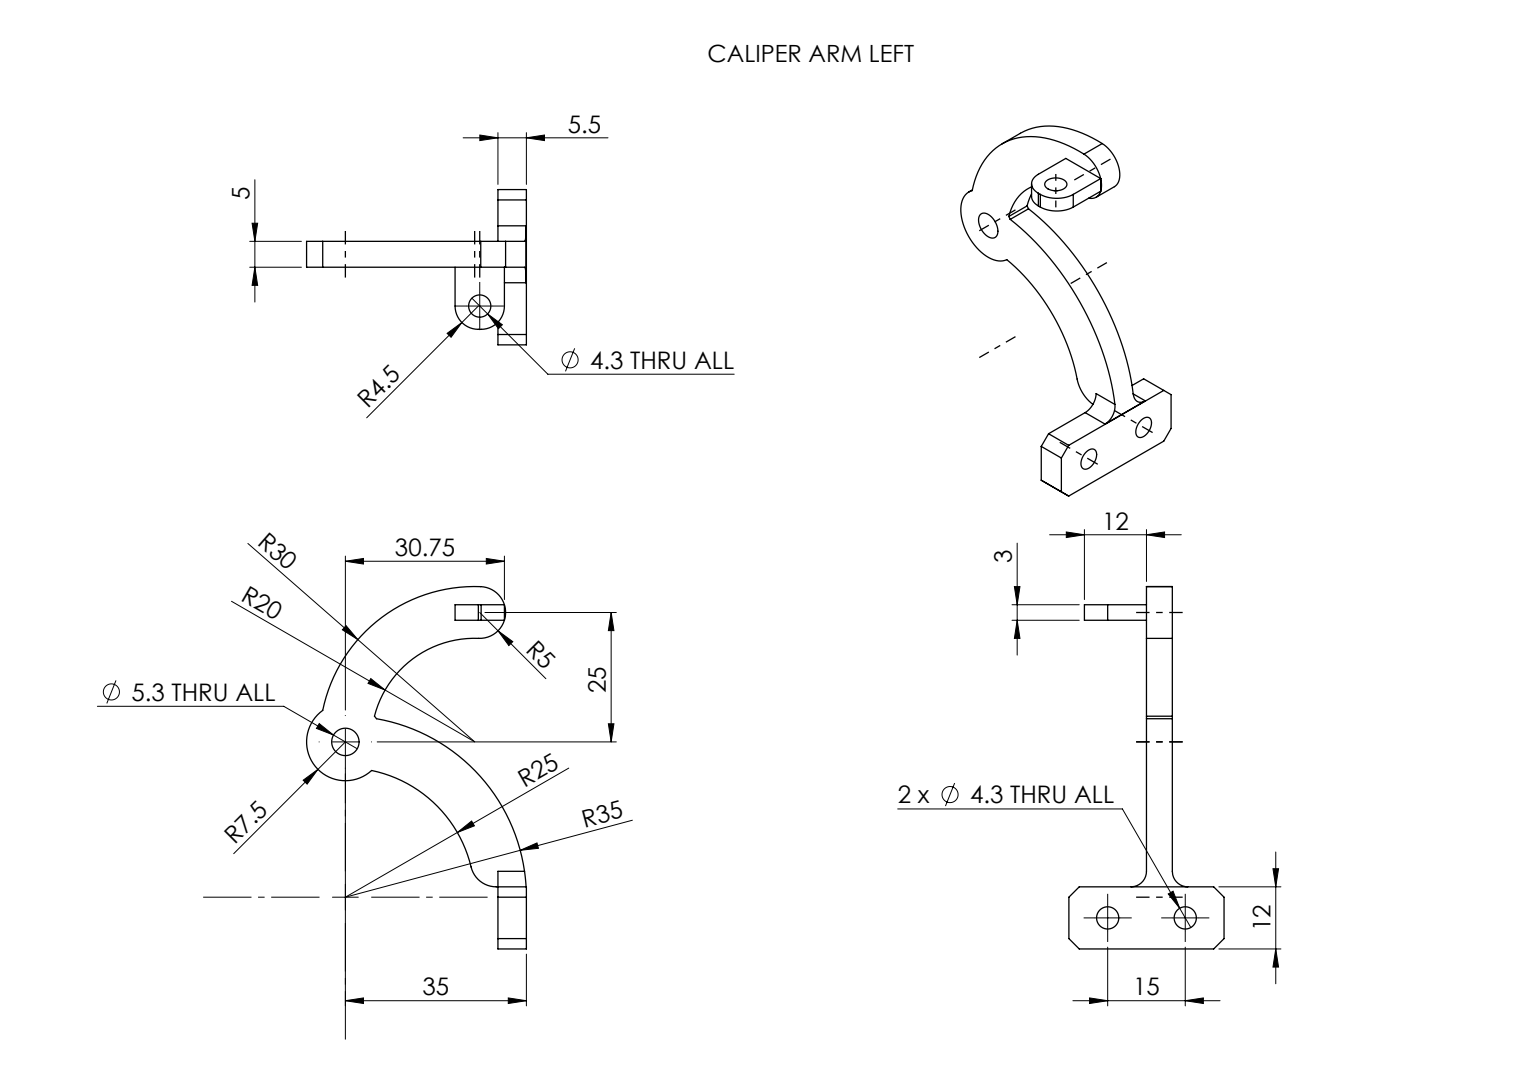
ISO-10303-21;
HEADER;
FILE_DESCRIPTION (('STEP AP214'),
    '1' );
FILE_NAME ('caliper arm left.step',
    '2026-10-08T05:45:04',
    ( '' ),
    ( '' ),
    'SwSTEP 2.0',
    'SolidWorks 2026',
    '' );
FILE_SCHEMA (( 'AUTOMOTIVE_DESIGN' ));
ENDSEC;

DATA;
#23=ADVANCED_FACE ( 'NONE', ( #9179, #3240, #3960 ), #10018, .T. ) ;
#34=CARTESIAN_POINT ( 'NONE',  ( 5.076455387921347651, 24.47916666666666075, -2.499999999999999112 ) ) ;
#40=VERTEX_POINT ( 'NONE', #10965 ) ;
#53=DIRECTION ( 'NONE',  ( 1.000000000000000000, 1.776356839400250465E-15, 0.000000000000000000 ) ) ;
#66=ORIENTED_EDGE ( 'NONE', *, *, #10280, .F. ) ;
#73=EDGE_CURVE ( 'NONE', #9208, #2549, #8067, .T. ) ;
#78=VECTOR ( 'NONE', #4837, 1000.000000000000000 ) ;
#79=DIRECTION ( 'NONE',  ( 0.000000000000000000, -1.000000000000000000, 0.000000000000000000 ) ) ;
#81=CARTESIAN_POINT ( 'NONE',  ( 29.50000000000000711, 1.387778780781445676E-14, -12.50000000000000000 ) ) ;
#86=CIRCLE ( 'NONE', #6829, 2.149999999999992362 ) ;
#90=EDGE_CURVE ( 'NONE', #5054, #1107, #1851, .T. ) ;
#96=ORIENTED_EDGE ( 'NONE', *, *, #10897, .F. ) ;
#98=EDGE_CURVE ( 'NONE', #7309, #1456, #9352, .T. ) ;
#99=FACE_OUTER_BOUND ( 'NONE', #8308, .T. ) ;
#100=AXIS2_PLACEMENT_3D ( 'NONE', #6064, #8518, #3293 ) ;
#102=CARTESIAN_POINT ( 'NONE',  ( 21.21106610644839208, 53.49999999999983658, 14.50000000000000000 ) ) ;
#108=EDGE_CURVE ( 'NONE', #2494, #2915, #8401, .T. ) ;
#112=CARTESIAN_POINT ( 'NONE',  ( 21.21106610644839208, 56.49999999999984368, 14.50000000000000000 ) ) ;
#113=EDGE_LOOP ( 'NONE', ( #698, #4129, #8999, #2220 ) ) ;
#127=DIRECTION ( 'NONE',  ( 0.000000000000000000, 0.000000000000000000, 1.000000000000000000 ) ) ;
#153=FACE_OUTER_BOUND ( 'NONE', #113, .T. ) ;
#156=ORIENTED_EDGE ( 'NONE', *, *, #2088, .F. ) ;
#176=PRESENTATION_STYLE_ASSIGNMENT (( #8567 ) ) ;
#183=VERTEX_POINT ( 'NONE', #900 ) ;
#202=CARTESIAN_POINT ( 'NONE',  ( 34.99999999999987210, -7.999999999999996447, -12.50000000000000000 ) ) ;
#208=ORIENTED_EDGE ( 'NONE', *, *, #385, .F. ) ;
#209=LINE ( 'NONE', #6940, #5064 ) ;
#217=LINE ( 'NONE', #1960, #6352 ) ;
#219=ORIENTED_EDGE ( 'NONE', *, *, #3408, .T. ) ;
#230=CARTESIAN_POINT ( 'NONE',  ( 34.99999999999987210, 2.000000000000002220, -12.50000000000000000 ) ) ;
#240=CARTESIAN_POINT ( 'NONE',  ( 6.015568632492061418, 34.47916666666664298, -2.499999999999998668 ) ) ;
#247=ORIENTED_EDGE ( 'NONE', *, *, #9284, .F. ) ;
#263=FACE_OUTER_BOUND ( 'NONE', #1330, .T. ) ;
#265=EDGE_LOOP ( 'NONE', ( #1963, #2238, #5184, #1794 ) ) ;
#277=LINE ( 'NONE', #2902, #2443 ) ;
#280=VECTOR ( 'NONE', #7293, 1000.000000000000000 ) ;
#284=CARTESIAN_POINT ( 'NONE',  ( 0.000000000000000000, 30.00000000000000000, 2.500000000000000000 ) ) ;
#289=PLANE ( 'NONE',  #436 ) ;
#290=DIRECTION ( 'NONE',  ( 0.000000000000000000, 1.000000000000000000, 0.000000000000000000 ) ) ;
#295=PLANE ( 'NONE',  #9853 ) ;
#302=EDGE_CURVE ( 'NONE', #8162, #681, #1693, .T. ) ;
#305=EDGE_CURVE ( 'NONE', #10997, #8894, #7125, .T. ) ;
#308=AXIS2_PLACEMENT_3D ( 'NONE', #6956, #4296, #9565 ) ;
#312=DIRECTION ( 'NONE',  ( -0.000000000000000000, 1.000000000000000000, -0.000000000000000000 ) ) ;
#320=CARTESIAN_POINT ( 'NONE',  ( 34.99999999999987210, -3.999999999999989786, 7.850000000000003197 ) ) ;
#322=ORIENTED_EDGE ( 'NONE', *, *, #302, .T. ) ;
#323=VECTOR ( 'NONE', #3846, 1000.000000000000114 ) ;
#355=DIRECTION ( 'NONE',  ( -6.098637220230966139E-17, 1.000000000000000000, 0.000000000000000000 ) ) ;
#371=CARTESIAN_POINT ( 'NONE',  ( 25.98076211353311749, 53.49999999999983658, 10.00000000000000178 ) ) ;
#373=AXIS2_PLACEMENT_3D ( 'NONE', #9911, #4914, #9286 ) ;
#377=ADVANCED_FACE ( 'NONE', ( #7914 ), #289, .T. ) ;
#379=ORIENTED_EDGE ( 'NONE', *, *, #4517, .F. ) ;
#381=VERTEX_POINT ( 'NONE', #2236 ) ;
#385=EDGE_CURVE ( 'NONE', #9319, #2915, #3021, .T. ) ;
#391=DIRECTION ( 'NONE',  ( 4.312387734422005941E-17, -0.7071067811865500152, 0.7071067811865451302 ) ) ;
#405=DIRECTION ( 'NONE',  ( -0.000000000000000000, -0.000000000000000000, -1.000000000000000000 ) ) ;
#410=DIRECTION ( 'NONE',  ( 1.000000000000000000, 0.000000000000000000, 0.000000000000000000 ) ) ;
#427=ORIENTED_EDGE ( 'NONE', *, *, #10489, .T. ) ;
#436=AXIS2_PLACEMENT_3D ( 'NONE', #3684, #4797, #8278 ) ;
#439=CIRCLE ( 'NONE', #9129, 7.500000000000000000 ) ;
#454=CARTESIAN_POINT ( 'NONE',  ( 24.99999259214812142, 30.01924558493218598, 2.500000000000000000 ) ) ;
#459=LINE ( 'NONE', #9638, #280 ) ;
#460=EDGE_CURVE ( 'NONE', #7106, #9208, #10799, .T. ) ;
#489=ORIENTED_EDGE ( 'NONE', *, *, #920, .T. ) ;
#492=AXIS2_PLACEMENT_3D ( 'NONE', #4378, #1817, #4149 ) ;
#498=EDGE_CURVE ( 'NONE', #8162, #10935, #5839, .T. ) ;
#500=EDGE_CURVE ( 'NONE', #2280, #1840, #8424, .T. ) ;
#505=CARTESIAN_POINT ( 'NONE',  ( 2.650000000000095834, 30.00000000000000000, -2.500000000000000000 ) ) ;
#506=ORIENTED_EDGE ( 'NONE', *, *, #5067, .T. ) ;
#524=EDGE_CURVE ( 'NONE', #2763, #4729, #7658, .T. ) ;
#529=DIRECTION ( 'NONE',  ( 1.000000000000000000, 0.000000000000000000, 0.000000000000000000 ) ) ;
#537=EDGE_LOOP ( 'NONE', ( #10892, #4237 ) ) ;
#542=ORIENTED_EDGE ( 'NONE', *, *, #9273, .T. ) ;
#558=AXIS2_PLACEMENT_3D ( 'NONE', #4552, #8823, #7936 ) ;
#565=ADVANCED_FACE ( 'NONE', ( #10231 ), #7677, .T. ) ;
#576=CARTESIAN_POINT ( 'NONE',  ( 30.75045812061784289, 53.49999999999983658, 14.50000000000000000 ) ) ;
#592=ORIENTED_EDGE ( 'NONE', *, *, #9149, .T. ) ;
#593=LINE ( 'NONE', #3109, #5602 ) ;
#606=CARTESIAN_POINT ( 'NONE',  ( 34.82492259089467979, 3.500278077966951340, -2.894288569839198022 ) ) ;
#607=LINE ( 'NONE', #3224, #5645 ) ;
#629=FACE_OUTER_BOUND ( 'NONE', #9860, .T. ) ;
#632=EDGE_CURVE ( 'NONE', #10983, #10935, #3603, .T. ) ;
#633=DIRECTION ( 'NONE',  ( 1.000000000000000000, -0.000000000000000000, -0.000000000000000000 ) ) ;
#658=CIRCLE ( 'NONE', #9718, 3.000000000000000000 ) ;
#679=ORIENTED_EDGE ( 'NONE', *, *, #9149, .F. ) ;
#681=VERTEX_POINT ( 'NONE', #6948 ) ;
#683=LINE ( 'NONE', #4766, #3461 ) ;
#684=PLANE ( 'NONE',  #6651 ) ;
#698=ORIENTED_EDGE ( 'NONE', *, *, #108, .F. ) ;
#701=PLANE ( 'NONE',  #10710 ) ;
#712=AXIS2_PLACEMENT_3D ( 'NONE', #9244, #9413, #4259 ) ;
#731=DIRECTION ( 'NONE',  ( -0.000000000000000000, 1.000000000000000000, -0.000000000000000000 ) ) ;
#738=DIRECTION ( 'NONE',  ( -0.000000000000000000, -0.000000000000000000, -1.000000000000000000 ) ) ;
#748=ORIENTED_EDGE ( 'NONE', *, *, #5542, .F. ) ;
#750=VERTEX_POINT ( 'NONE', #7844 ) ;
#758=DIRECTION ( 'NONE',  ( -1.000000000000000000, 0.000000000000000000, 0.000000000000000000 ) ) ;
#776=CARTESIAN_POINT ( 'NONE',  ( 29.50000000000000711, -3.999999999999989786, -2.850000000000007194 ) ) ;
#786=CIRCLE ( 'NONE', #10023, 2.649999999999992362 ) ;
#788=VECTOR ( 'NONE', #2505, 1000.000000000000000 ) ;
#796=CARTESIAN_POINT ( 'NONE',  ( 25.71106610644839208, 53.49999999999983658, 14.50000000000000000 ) ) ;
#823=EDGE_CURVE ( 'NONE', #8525, #1015, #3146, .T. ) ;
#826=CYLINDRICAL_SURFACE ( 'NONE', #6009, 7.500000000000000000 ) ;
#830=CARTESIAN_POINT ( 'NONE',  ( 6.098637220230963427E-16, -10.00000000000000000, 0.000000000000000000 ) ) ;
#832=ORIENTED_EDGE ( 'NONE', *, *, #10941, .F. ) ;
#841=AXIS2_PLACEMENT_3D ( 'NONE', #5509, #10615, #4675 ) ;
#842=COLOUR_RGB ( '', 0.72549020, 0.75294118, 0.79215686) ;
#847=DIRECTION ( 'NONE',  ( -1.000000000000000000, -6.098637220230963674E-17, 0.000000000000000000 ) ) ;
#852=CYLINDRICAL_SURFACE ( 'NONE', #1893, 2.149999999999988809 ) ;
#858=CARTESIAN_POINT ( 'NONE',  ( 34.90196196521935690, 2.620161469061431880, 3.662783066803843468 ) ) ;
#861=CARTESIAN_POINT ( 'NONE',  ( 34.99999999999987210, -9.999999999999998224, -10.50000000000001243 ) ) ;
#867=EDGE_CURVE ( 'NONE', #9108, #1634, #6971, .T. ) ;
#874=VERTEX_POINT ( 'NONE', #8674 ) ;
#891=ORIENTED_EDGE ( 'NONE', *, *, #7285, .T. ) ;
#900=CARTESIAN_POINT ( 'NONE',  ( 25.98076211353311749, 56.49999999999984368, 7.850000000000009415 ) ) ;
#905=EDGE_CURVE ( 'NONE', #7610, #10564, #3067, .T. ) ;
#916=EDGE_LOOP ( 'NONE', ( #9339, #3984, #219, #3158 ) ) ;
#917=CARTESIAN_POINT ( 'NONE',  ( 29.50000000000000711, -7.999999999999996447, -12.50000000000000000 ) ) ;
#918=CARTESIAN_POINT ( 'NONE',  ( 34.99999999999987210, 2.000000000000002220, -10.49999999999999822 ) ) ;
#920=EDGE_CURVE ( 'NONE', #7348, #750, #2720, .T. ) ;
#924=DIRECTION ( 'NONE',  ( 1.000000000000000000, -0.000000000000000000, -0.000000000000000000 ) ) ;
#926=VECTOR ( 'NONE', #5218, 1000.000000000000114 ) ;
#934=FACE_OUTER_BOUND ( 'NONE', #7050, .T. ) ;
#935=DIRECTION ( 'NONE',  ( -0.000000000000000000, -0.000000000000000000, -1.000000000000000000 ) ) ;
#953=EDGE_CURVE ( 'NONE', #1015, #6697, #6053, .T. ) ;
#955=CARTESIAN_POINT ( 'NONE',  ( -1.219727444046192735E-16, 2.000000000000000000, -10.49999999999999822 ) ) ;
#972=FILL_AREA_STYLE ('',( #1601 ) ) ;
#973=AXIS2_PLACEMENT_3D ( 'NONE', #3761, #312, #4606 ) ;
#975=VECTOR ( 'NONE', #847, 1000.000000000000000 ) ;
#983=CARTESIAN_POINT ( 'NONE',  ( 34.99999999999987210, 2.000000000000002220, 15.49999999999999645 ) ) ;
#992=AXIS2_PLACEMENT_3D ( 'NONE', #9238, #4978, #5147 ) ;
#1003=ORIENTED_EDGE ( 'NONE', *, *, #8256, .T. ) ;
#1012=DIRECTION ( 'NONE',  ( 1.000000000000000000, -2.212882687011047826E-16, 0.000000000000000000 ) ) ;
#1015=VERTEX_POINT ( 'NONE', #6180 ) ;
#1016=LINE ( 'NONE', #10524, #1355 ) ;
#1018=AXIS2_PLACEMENT_3D ( 'NONE', #830, #6007, #6951 ) ;
#1037=DIRECTION ( 'NONE',  ( 2.212882687011047826E-16, 1.000000000000000000, -0.000000000000000000 ) ) ;
#1043=CARTESIAN_POINT ( 'NONE',  ( 34.99999999999987210, 1.431146867680865853E-14, -12.50000000000000000 ) ) ;
#1044=PRODUCT_CONTEXT ( 'NONE', #7789, 'mechanical' ) ;
#1053=ORIENTED_EDGE ( 'NONE', *, *, #9284, .T. ) ;
#1055=ORIENTED_EDGE ( 'NONE', *, *, #8721, .T. ) ;
#1057=ORIENTED_EDGE ( 'NONE', *, *, #6360, .T. ) ;
#1076=LINE ( 'NONE', #10587, #10450 ) ;
#1083=CARTESIAN_POINT ( 'NONE',  ( -3.049318610115482207E-16, 5.000000000000000000, 5.500000000000000000 ) ) ;
#1085=FACE_OUTER_BOUND ( 'NONE', #3210, .T. ) ;
#1092=EDGE_CURVE ( 'NONE', #1254, #8525, #5107, .T. ) ;
#1093=VERTEX_POINT ( 'NONE', #34 ) ;
#1094=CARTESIAN_POINT ( 'NONE',  ( 30.75045812061784289, 53.49999999999983658, 2.500000000000000000 ) ) ;
#1098=DIRECTION ( 'NONE',  ( 0.000000000000000000, 1.000000000000000000, 0.000000000000000000 ) ) ;
#1104=ADVANCED_FACE ( 'NONE', ( #153 ), #7714, .F. ) ;
#1107=VERTEX_POINT ( 'NONE', #3319 ) ;
#1108=DIRECTION ( 'NONE',  ( 6.098637220230963674E-17, -1.000000000000000000, 0.000000000000000000 ) ) ;
#1111=VECTOR ( 'NONE', #4090, 1000.000000000000000 ) ;
#1114=( LENGTH_UNIT ( ) NAMED_UNIT ( * ) SI_UNIT ( .MILLI., .METRE. ) );
#1120=DIRECTION ( 'NONE',  ( 0.000000000000000000, 0.000000000000000000, -1.000000000000000000 ) ) ;
#1123=ORIENTED_EDGE ( 'NONE', *, *, #4241, .F. ) ;
#1132=CARTESIAN_POINT ( 'NONE',  ( 34.94281041931228771, 2.000000000000002220, 2.500000000000000000 ) ) ;
#1133=CIRCLE ( 'NONE', #8225, 4.999999999999997335 ) ;
#1134=ORIENTED_EDGE ( 'NONE', *, *, #5268, .F. ) ;
#1141=CYLINDRICAL_SURFACE ( 'NONE', #973, 2.149999999999988809 ) ;
#1143=DIRECTION ( 'NONE',  ( -0.000000000000000000, 1.000000000000000000, -0.000000000000000000 ) ) ;
#1145=AXIS2_PLACEMENT_3D ( 'NONE', #6201, #9587, #410 ) ;
#1149=CIRCLE ( 'NONE', #5763, 2.149999999999988809 ) ;
#1154=CARTESIAN_POINT ( 'NONE',  ( 34.99999999999987210, 1.431146867680865853E-14, 17.49999999999999645 ) ) ;
#1156=DIRECTION ( 'NONE',  ( 0.000000000000000000, -1.000000000000000000, 0.000000000000000000 ) ) ;
#1163=ORIENTED_EDGE ( 'NONE', *, *, #6957, .T. ) ;
#1167=VECTOR ( 'NONE', #6619, 1000.000000000000000 ) ;
#1179=EDGE_CURVE ( 'NONE', #681, #3312, #8596, .T. ) ;
#1180=ORIENTED_EDGE ( 'NONE', *, *, #8476, .T. ) ;
#1202=EDGE_CURVE ( 'NONE', #6168, #6073, #6594, .T. ) ;
#1206=CARTESIAN_POINT ( 'NONE',  ( 34.99999999999987210, -9.999999999999998224, 15.49999999999998934 ) ) ;
#1207=VECTOR ( 'NONE', #9723, 1000.000000000000000 ) ;
#1209=LINE ( 'NONE', #7937, #5883 ) ;
#1224=ORIENTED_EDGE ( 'NONE', *, *, #5136, .F. ) ;
#1237=CARTESIAN_POINT ( 'NONE',  ( 21.21106610644839208, 53.49999999999983658, 14.50000000000000000 ) ) ;
#1253=CARTESIAN_POINT ( 'NONE',  ( 29.50000000000000711, -3.999999999999989786, 9.999999999999998224 ) ) ;
#1254=VERTEX_POINT ( 'NONE', #983 ) ;
#1281=ORIENTED_EDGE ( 'NONE', *, *, #1179, .T. ) ;
#1295=EDGE_LOOP ( 'NONE', ( #8009, #4620, #5332, #9406 ) ) ;
#1298=CYLINDRICAL_SURFACE ( 'NONE', #5272, 2.649999999999991029 ) ;
#1305=CARTESIAN_POINT ( 'NONE',  ( 21.21106610644839208, 56.49999999999984368, 14.50000000000000000 ) ) ;
#1307=LINE ( 'NONE', #3915, #5108 ) ;
#1309=CYLINDRICAL_SURFACE ( 'NONE', #5601, 3.000000000000000000 ) ;
#1314=VECTOR ( 'NONE', #2944, 1000.000000000000000 ) ;
#1315=DIRECTION ( 'NONE',  ( 0.000000000000000000, -1.000000000000000000, 0.000000000000000000 ) ) ;
#1323=ORIENTED_EDGE ( 'NONE', *, *, #3560, .T. ) ;
#1324=EDGE_CURVE ( 'NONE', #4849, #2261, #6962, .T. ) ;
#1325=CARTESIAN_POINT ( 'NONE',  ( 34.94281041931228771, 5.000000000000001776, 2.500000000000000000 ) ) ;
#1327=VECTOR ( 'NONE', #7145, 1000.000000000000000 ) ;
#1330=EDGE_LOOP ( 'NONE', ( #5656, #4328, #8187, #2492 ) ) ;
#1336=AXIS2_PLACEMENT_3D ( 'NONE', #5007, #8382, #758 ) ;
#1337=ORIENTED_EDGE ( 'NONE', *, *, #10941, .T. ) ;
#1354=EDGE_CURVE ( 'NONE', #183, #9110, #8369, .T. ) ;
#1355=VECTOR ( 'NONE', #9627, 1000.000000000000000 ) ;
#1373=LINE ( 'NONE', #576, #5611 ) ;
#1375=PRODUCT_DEFINITION ( 'UNKNOWN', '', #7225, #8335 ) ;
#1376=CIRCLE ( 'NONE', #5462, 2.149999999999992362 ) ;
#1384=VECTOR ( 'NONE', #5130, 1000.000000000000000 ) ;
#1402=EDGE_CURVE ( 'NONE', #6697, #1254, #6987, .T. ) ;
#1404=CARTESIAN_POINT ( 'NONE',  ( 34.94281041931228771, 2.000000000000002665, -5.301324476612966130 ) ) ;
#1413=CARTESIAN_POINT ( 'NONE',  ( 21.21106610644839208, 56.49999999999984368, 2.500000000000000000 ) ) ;
#1415=DIRECTION ( 'NONE',  ( -0.000000000000000000, 0.000000000000000000, 1.000000000000000000 ) ) ;
#1436=UNCERTAINTY_MEASURE_WITH_UNIT (LENGTH_MEASURE( 1.000000000000000082E-05 ), #6013, 'distance_accuracy_value', 'NONE');
#1437=VERTEX_POINT ( 'NONE', #7881 ) ;
#1445=ORIENTED_EDGE ( 'NONE', *, *, #6596, .F. ) ;
#1449=EDGE_CURVE ( 'NONE', #7957, #3879, #3596, .T. ) ;
#1453=DIRECTION ( 'NONE',  ( 1.000000000000000000, -0.000000000000000000, -0.000000000000000000 ) ) ;
#1456=VERTEX_POINT ( 'NONE', #1206 ) ;
#1462=CARTESIAN_POINT ( 'NONE',  ( 34.64101615137754919, 5.000000000000002665, 2.500000000000000000 ) ) ;
#1469=ORIENTED_EDGE ( 'NONE', *, *, #9598, .F. ) ;
#1471=LINE ( 'NONE', #10802, #4745 ) ;
#1493=VERTEX_POINT ( 'NONE', #5806 ) ;
#1503=CARTESIAN_POINT ( 'NONE',  ( 34.69578914996070296, 4.608685395970379517, -2.519144107514304398 ) ) ;
#1510=VECTOR ( 'NONE', #4752, 1000.000000000000000 ) ;
#1526=DIRECTION ( 'NONE',  ( 1.000000000000000000, 0.000000000000000000, 0.000000000000000000 ) ) ;
#1532=CARTESIAN_POINT ( 'NONE',  ( 5.621179405865835754, 34.96511249490581008, 2.500000000000000000 ) ) ;
#1554=AXIS2_PLACEMENT_3D ( 'NONE', #2026, #4533, #9634 ) ;
#1563=ORIENTED_EDGE ( 'NONE', *, *, #6544, .T. ) ;
#1571=CARTESIAN_POINT ( 'NONE',  ( 29.50000000000000711, 2.000000000000001776, 2.500000000000000444 ) ) ;
#1575=EDGE_LOOP ( 'NONE', ( #5448, #9550, #1180, #4570 ) ) ;
#1584=CARTESIAN_POINT ( 'NONE',  ( 34.92403196580097813, 2.306010598194981664, 4.165547504151214220 ) ) ;
#1592=LINE ( 'NONE', #10985, #9194 ) ;
#1601=FILL_AREA_STYLE_COLOUR ( '', #8306 ) ;
#1603=EDGE_LOOP ( 'NONE', ( #4104, #1053, #1842, #4564 ) ) ;
#1607=EDGE_LOOP ( 'NONE', ( #4800, #10163, #96, #4089, #10341, #4390, #748, #2683, #7548, #10701, #1055 ) ) ;
#1610=CYLINDRICAL_SURFACE ( 'NONE', #1336, 4.999999999999997335 ) ;
#1619=ORIENTED_EDGE ( 'NONE', *, *, #823, .T. ) ;
#1632=DIRECTION ( 'NONE',  ( 4.312387734421997929E-17, -0.7071067811865487940, -0.7071067811865463515 ) ) ;
#1634=VERTEX_POINT ( 'NONE', #6749 ) ;
#1635=ORIENTED_EDGE ( 'NONE', *, *, #7169, .F. ) ;
#1648=DIRECTION ( 'NONE',  ( 1.000000000000000000, -9.251858538542971828E-16, 0.000000000000000000 ) ) ;
#1656=ORIENTED_EDGE ( 'NONE', *, *, #3408, .F. ) ;
#1657=DIRECTION ( 'NONE',  ( 0.000000000000000000, -1.000000000000000000, 0.000000000000000000 ) ) ;
#1662=VERTEX_POINT ( 'NONE', #796 ) ;
#1664=DIRECTION ( 'NONE',  ( -1.000000000000000000, -6.098637220230963674E-17, 0.000000000000000000 ) ) ;
#1682=VECTOR ( 'NONE', #1012, 1000.000000000000000 ) ;
#1693=CIRCLE ( 'NONE', #7367, 4.500000000000000000 ) ;
#1702=VECTOR ( 'NONE', #2138, 1000.000000000000000 ) ;
#1718=CARTESIAN_POINT ( 'NONE',  ( 0.000000000000000000, 30.00000000000000000, -2.499999999999998668 ) ) ;
#1753=ADVANCED_FACE ( 'NONE', ( #4316 ), #5917, .T. ) ;
#1765=DIRECTION ( 'NONE',  ( -1.000000000000000000, -6.098637220230963674E-17, 0.000000000000000000 ) ) ;
#1766=ORIENTED_EDGE ( 'NONE', *, *, #2279, .F. ) ;
#1767=LINE ( 'NONE', #917, #7339 ) ;
#1782=FACE_OUTER_BOUND ( 'NONE', #1603, .T. ) ;
#1794=ORIENTED_EDGE ( 'NONE', *, *, #3531, .F. ) ;
#1805=EDGE_CURVE ( 'NONE', #10564, #183, #7190, .T. ) ;
#1815=LINE ( 'NONE', #7089, #3829 ) ;
#1816=ORIENTED_EDGE ( 'NONE', *, *, #10153, .F. ) ;
#1817=DIRECTION ( 'NONE',  ( 0.000000000000000000, -0.000000000000000000, -1.000000000000000000 ) ) ;
#1823=CARTESIAN_POINT ( 'NONE',  ( 30.75045812061784289, 56.49999999999984368, 14.50000000000000000 ) ) ;
#1832=EDGE_CURVE ( 'NONE', #7103, #7090, #1076, .T. ) ;
#1833=DIRECTION ( 'NONE',  ( 0.000000000000000000, 0.000000000000000000, -1.000000000000000000 ) ) ;
#1835=CARTESIAN_POINT ( 'NONE',  ( 34.64101615137754919, 5.000000000000002665, -2.500000000000000000 ) ) ;
#1840=VERTEX_POINT ( 'NONE', #8643 ) ;
#1841=FACE_OUTER_BOUND ( 'NONE', #10523, .T. ) ;
#1842=ORIENTED_EDGE ( 'NONE', *, *, #524, .F. ) ;
#1851=LINE ( 'NONE', #955, #975 ) ;
#1852=DIRECTION ( 'NONE',  ( 0.000000000000000000, 1.000000000000000000, 0.000000000000000000 ) ) ;
#1855=ORIENTED_EDGE ( 'NONE', *, *, #7793, .F. ) ;
#1869=( NAMED_UNIT ( * ) SI_UNIT ( $, .STERADIAN. ) SOLID_ANGLE_UNIT ( ) );
#1872=VECTOR ( 'NONE', #7281, 1000.000000000000000 ) ;
#1885=ORIENTED_EDGE ( 'NONE', *, *, #5967, .F. ) ;
#1892=PLANE ( 'NONE',  #4534 ) ;
#1893=AXIS2_PLACEMENT_3D ( 'NONE', #10249, #731, #2411 ) ;
#1909=FILL_AREA_STYLE ('',( #10293 ) ) ;
#1913=CARTESIAN_POINT ( 'NONE',  ( 29.50000000000000711, -7.999999999999996447, -12.50000000000000000 ) ) ;
#1919=PLANE ( 'NONE',  #4194 ) ;
#1933=CIRCLE ( 'NONE', #492, 20.00000000000000355 ) ;
#1937=ADVANCED_FACE ( 'NONE', ( #9856 ), #8080, .T. ) ;
#1951=VERTEX_POINT ( 'NONE', #1413 ) ;
#1954=ADVANCED_FACE ( 'NONE', ( #4806 ), #826, .T. ) ;
#1956=DIRECTION ( 'NONE',  ( 0.000000000000000000, 0.000000000000000000, 1.000000000000000000 ) ) ;
#1960=CARTESIAN_POINT ( 'NONE',  ( 29.50000000000000711, 2.000000000000001776, -12.50000000000000000 ) ) ;
#1963=ORIENTED_EDGE ( 'NONE', *, *, #2382, .F. ) ;
#1973=FACE_OUTER_BOUND ( 'NONE', #8882, .T. ) ;
#1993=ORIENTED_EDGE ( 'NONE', *, *, #1324, .T. ) ;
#1997=DIRECTION ( 'NONE',  ( 1.000000000000000000, -0.000000000000000000, -0.000000000000000000 ) ) ;
#2018=PLANE ( 'NONE',  #10066 ) ;
#2023=LINE ( 'NONE', #9746, #1702 ) ;
#2026=CARTESIAN_POINT ( 'NONE',  ( 0.000000000000000000, 0.000000000000000000, -2.500000000000000000 ) ) ;
#2033=CARTESIAN_POINT ( 'NONE',  ( 34.99999999999987210, 2.000000000000002220, 17.49999999999999645 ) ) ;
#2045=ORIENTED_EDGE ( 'NONE', *, *, #4707, .F. ) ;
#2056=EDGE_CURVE ( 'NONE', #3381, #7103, #2651, .T. ) ;
#2088=EDGE_CURVE ( 'NONE', #1662, #10997, #5832, .T. ) ;
#2098=PLANE ( 'NONE',  #3491 ) ;
#2103=PRODUCT_DEFINITION_SHAPE ( 'NONE', 'NONE',  #1375 ) ;
#2114=VECTOR ( 'NONE', #6232, 1000.000000000000000 ) ;
#2116=CARTESIAN_POINT ( 'NONE',  ( 25.71106610644839208, 0.000000000000000000, 14.50000000000000000 ) ) ;
#2138=DIRECTION ( 'NONE',  ( -1.000000000000000000, -6.098637220230963674E-17, -0.000000000000000000 ) ) ;
#2139=DIRECTION ( 'NONE',  ( 1.000000000000000000, 0.000000000000000000, 0.000000000000000000 ) ) ;
#2150=CARTESIAN_POINT ( 'NONE',  ( 0.000000000000000000, 0.000000000000000000, 2.500000000000000000 ) ) ;
#2169=DIRECTION ( 'NONE',  ( 1.000000000000000000, 0.000000000000000000, 0.000000000000000000 ) ) ;
#2178=AXIS2_PLACEMENT_3D ( 'NONE', #9556, #8722, #1956 ) ;
#2179=CARTESIAN_POINT ( 'NONE',  ( 34.91794119163850496, 2.397787035234373310, -3.994322637888108485 ) ) ;
#2181=ORIENTED_EDGE ( 'NONE', *, *, #2382, .T. ) ;
#2182=ORIENTED_EDGE ( 'NONE', *, *, #6710, .F. ) ;
#2189=DIRECTION ( 'NONE',  ( 0.000000000000000000, -1.000000000000000000, 0.000000000000000000 ) ) ;
#2194=DIRECTION ( 'NONE',  ( -0.000000000000000000, -1.000000000000000000, -0.000000000000000000 ) ) ;
#2196=CARTESIAN_POINT ( 'NONE',  ( 29.50000000000000711, 2.000000000000001776, 5.500000000000001776 ) ) ;
#2200=VECTOR ( 'NONE', #6936, 1000.000000000000000 ) ;
#2204=ORIENTED_EDGE ( 'NONE', *, *, #6466, .T. ) ;
#2211=ADVANCED_FACE ( 'NONE', ( #10845 ), #8343, .F. ) ;
#2218=EDGE_CURVE ( 'NONE', #5054, #1254, #6733, .T. ) ;
#2220=ORIENTED_EDGE ( 'NONE', *, *, #3035, .F. ) ;
#2236=CARTESIAN_POINT ( 'NONE',  ( 34.94281041931228771, 2.000000000000002220, 5.500000000000000000 ) ) ;
#2238=ORIENTED_EDGE ( 'NONE', *, *, #8447, .F. ) ;
#2250=EDGE_LOOP ( 'NONE', ( #9722, #6708, #2722, #208, #9563, #2628, #427, #9652, #10160, #1123, #3401, #7607, #9046, #2783, #2836 ) ) ;
#2261=VERTEX_POINT ( 'NONE', #776 ) ;
#2274=ORIENTED_EDGE ( 'NONE', *, *, #6710, .T. ) ;
#2279=EDGE_CURVE ( 'NONE', #6762, #2549, #5527, .T. ) ;
#2280=VERTEX_POINT ( 'NONE', #3294 ) ;
#2283=LINE ( 'NONE', #2440, #78 ) ;
#2332=CARTESIAN_POINT ( 'NONE',  ( 29.50000000000000711, 1.387778780781445676E-14, 17.49999999999999645 ) ) ;
#2336=CARTESIAN_POINT ( 'NONE',  ( 34.76713615931384993, 4.034733667027952997, -2.652855901285304796 ) ) ;
#2344=CARTESIAN_POINT ( 'NONE',  ( 34.74418829745650328, 4.228279689541293962, 2.594445730714923126 ) ) ;
#2356=FACE_OUTER_BOUND ( 'NONE', #2946, .T. ) ;
#2363=ORIENTED_EDGE ( 'NONE', *, *, #4819, .F. ) ;
#2382=EDGE_CURVE ( 'NONE', #6022, #381, #7696, .T. ) ;
#2385=DIRECTION ( 'NONE',  ( 1.000000000000000000, 0.000000000000000000, 0.000000000000000000 ) ) ;
#2392=VECTOR ( 'NONE', #1632, 1000.000000000000000 ) ;
#2410=EDGE_LOOP ( 'NONE', ( #2733, #5468, #10851, #4676 ) ) ;
#2411=DIRECTION ( 'NONE',  ( 0.000000000000000000, 0.000000000000000000, 1.000000000000000000 ) ) ;
#2412=AXIS2_PLACEMENT_3D ( 'NONE', #9025, #1415, #4808 ) ;
#2419=CARTESIAN_POINT ( 'NONE',  ( 34.94281041931228771, 2.000000000000002220, 5.500000000000000000 ) ) ;
#2435=ADVANCED_FACE ( 'NONE', ( #10143 ), #10916, .F. ) ;
#2440=CARTESIAN_POINT ( 'NONE',  ( 21.21106610644839208, 53.49999999999983658, 14.50000000000000000 ) ) ;
#2443=VECTOR ( 'NONE', #8893, 1000.000000000000000 ) ;
#2445=AXIS2_PLACEMENT_3D ( 'NONE', #8555, #4162, #2385 ) ;
#2452=MECHANICAL_DESIGN_GEOMETRIC_PRESENTATION_REPRESENTATION('',(#4953),#5300);
#2456=LINE ( 'NONE', #505, #5292 ) ;
#2492=ORIENTED_EDGE ( 'NONE', *, *, #6360, .F. ) ;
#2494=VERTEX_POINT ( 'NONE', #4136 ) ;
#2497=ORIENTED_EDGE ( 'NONE', *, *, #5677, .F. ) ;
#2505=DIRECTION ( 'NONE',  ( -1.000000000000000000, -0.000000000000000000, -0.000000000000000000 ) ) ;
#2529=UNCERTAINTY_MEASURE_WITH_UNIT (LENGTH_MEASURE( 1.000000000000000082E-05 ), #1114, 'distance_accuracy_value', 'NONE');
#2542=EDGE_CURVE ( 'NONE', #7103, #3195, #2874, .T. ) ;
#2549=VERTEX_POINT ( 'NONE', #240 ) ;
#2552=ORIENTED_EDGE ( 'NONE', *, *, #73, .T. ) ;
#2556=DIRECTION ( 'NONE',  ( 0.000000000000000000, 0.000000000000000000, 1.000000000000000000 ) ) ;
#2584=ORIENTED_EDGE ( 'NONE', *, *, #1092, .F. ) ;
#2586=ORIENTED_EDGE ( 'NONE', *, *, #90, .T. ) ;
#2588=VECTOR ( 'NONE', #2556, 1000.000000000000000 ) ;
#2624=CARTESIAN_POINT ( 'NONE',  ( 1.047444401652940007E-13, 30.00000000000000000, -2.500000000000000000 ) ) ;
#2628=ORIENTED_EDGE ( 'NONE', *, *, #8772, .T. ) ;
#2644=DIRECTION ( 'NONE',  ( -0.000000000000000000, 0.000000000000000000, 1.000000000000000000 ) ) ;
#2651=CIRCLE ( 'NONE', #8852, 20.00000000000000355 ) ;
#2670=DIRECTION ( 'NONE',  ( 1.000000000000000000, 0.000000000000000000, 0.000000000000000000 ) ) ;
#2680=CARTESIAN_POINT ( 'NONE',  ( 24.99999259214812142, 30.01924558493218598, 2.500000000000000000 ) ) ;
#2683=ORIENTED_EDGE ( 'NONE', *, *, #2279, .T. ) ;
#2710=ORIENTED_EDGE ( 'NONE', *, *, #6636, .F. ) ;
#2714=AXIS2_PLACEMENT_3D ( 'NONE', #3816, #1143, #2883 ) ;
#2718=CARTESIAN_POINT ( 'NONE',  ( 34.99999999999987210, -3.999999999999989786, -4.999999999999999112 ) ) ;
#2720=CIRCLE ( 'NONE', #6422, 2.649999999999992362 ) ;
#2722=ORIENTED_EDGE ( 'NONE', *, *, #108, .T. ) ;
#2733=ORIENTED_EDGE ( 'NONE', *, *, #1179, .F. ) ;
#2755=CIRCLE ( 'NONE', #1145, 35.00000000000000000 ) ;
#2763=VERTEX_POINT ( 'NONE', #3076 ) ;
#2770=CIRCLE ( 'NONE', #7047, 30.00000000000000000 ) ;
#2774=DIRECTION ( 'NONE',  ( -0.000000000000000000, 0.000000000000000000, 1.000000000000000000 ) ) ;
#2778=VECTOR ( 'NONE', #9473, 1000.000000000000000 ) ;
#2783=ORIENTED_EDGE ( 'NONE', *, *, #5002, .F. ) ;
#2789=CARTESIAN_POINT ( 'NONE',  ( 25.98076211353311749, 53.49999999999983658, 10.00000000000000178 ) ) ;
#2800=LINE ( 'NONE', #9618, #9007 ) ;
#2804=CARTESIAN_POINT ( 'NONE',  ( 29.17190429162964094, 2.000000000000001776, 17.50099999999999767 ) ) ;
#2806=VECTOR ( 'NONE', #8913, 1000.000000000000000 ) ;
#2825=AXIS2_PLACEMENT_3D ( 'NONE', #1083, #7823, #355 ) ;
#2829=CARTESIAN_POINT ( 'NONE',  ( -1.219727444046192735E-16, 2.000000000000000000, 0.000000000000000000 ) ) ;
#2836=ORIENTED_EDGE ( 'NONE', *, *, #8107, .T. ) ;
#2839=DIRECTION ( 'NONE',  ( 4.312387734421975743E-17, -0.7071067811865451302, -0.7071067811865500152 ) ) ;
#2840=ADVANCED_BREP_SHAPE_REPRESENTATION ( '', ( #5541, #308 ), #10083 ) ;
#2857=CARTESIAN_POINT ( 'NONE',  ( 29.17190429162964094, 7.000000000000002665, -2.500000000000000000 ) ) ;
#2865=FACE_OUTER_BOUND ( 'NONE', #2250, .T. ) ;
#2874=CIRCLE ( 'NONE', #712, 4.999999999999997335 ) ;
#2883=DIRECTION ( 'NONE',  ( 0.000000000000000000, 0.000000000000000000, 1.000000000000000000 ) ) ;
#2885=ORIENTED_EDGE ( 'NONE', *, *, #953, .T. ) ;
#2894=DIRECTION ( 'NONE',  ( 1.000000000000000000, 6.098637220230963674E-17, -0.000000000000000000 ) ) ;
#2902=CARTESIAN_POINT ( 'NONE',  ( 26.25045812061784289, 0.000000000000000000, 14.50000000000000000 ) ) ;
#2905=ORIENTED_EDGE ( 'NONE', *, *, #8772, .F. ) ;
#2914=DIRECTION ( 'NONE',  ( 1.000000000000000000, 6.098637220230963674E-17, 0.000000000000000000 ) ) ;
#2915=VERTEX_POINT ( 'NONE', #1571 ) ;
#2916=EDGE_LOOP ( 'NONE', ( #2274, #7235, #8984, #4264, #6768, #2885, #7111, #10354, #3084, #7563, #6085, #1163, #1003, #4364 ) ) ;
#2918=DIRECTION ( 'NONE',  ( 1.000000000000000000, 0.000000000000000000, 0.000000000000000000 ) ) ;
#2930=LINE ( 'NONE', #2033, #4032 ) ;
#2935=AXIS2_PLACEMENT_3D ( 'NONE', #1718, #9488, #8378 ) ;
#2944=DIRECTION ( 'NONE',  ( 0.000000000000000000, 1.000000000000000000, 0.000000000000000000 ) ) ;
#2946=EDGE_LOOP ( 'NONE', ( #2552, #5823, #2905, #2181, #1323, #5683 ) ) ;
#2988=AXIS2_PLACEMENT_3D ( 'NONE', #10784, #1453, #5680 ) ;
#3000=EDGE_LOOP ( 'NONE', ( #9977, #1656, #1469, #5840, #10769, #4986 ) ) ;
#3003=AXIS2_PLACEMENT_3D ( 'NONE', #9371, #3431, #6806 ) ;
#3016=SHAPE_REPRESENTATION ( 'caliper arm left', ( #308 ), #10083 ) ;
#3021=LINE ( 'NONE', #10001, #1872 ) ;
#3024=VERTEX_POINT ( 'NONE', #1913 ) ;
#3030=CARTESIAN_POINT ( 'NONE',  ( 0.000000000000000000, 30.00000000000000000, -23.71320343559643007 ) ) ;
#3035=EDGE_CURVE ( 'NONE', #2915, #40, #1209, .T. ) ;
#3037=CARTESIAN_POINT ( 'NONE',  ( 30.75045812061784289, 53.49999999999983658, 10.00000000000000178 ) ) ;
#3063=AXIS2_PLACEMENT_3D ( 'NONE', #2718, #924, #6874 ) ;
#3067=CIRCLE ( 'NONE', #6078, 2.149999999999988809 ) ;
#3068=CARTESIAN_POINT ( 'NONE',  ( 34.94281041931228771, 2.000000000000002220, -5.500000000000000000 ) ) ;
#3069=DIRECTION ( 'NONE',  ( 1.000000000000000000, 6.098637220230963674E-17, 0.000000000000000000 ) ) ;
#3076=CARTESIAN_POINT ( 'NONE',  ( 5.076455387921339657, 24.47916666666667140, 2.500000000000000000 ) ) ;
#3084=ORIENTED_EDGE ( 'NONE', *, *, #385, .T. ) ;
#3097=CARTESIAN_POINT ( 'NONE',  ( 2.650000000000097167, 30.00000000000000000, -2.500000000000000000 ) ) ;
#3107=ORIENTED_EDGE ( 'NONE', *, *, #1092, .T. ) ;
#3109=CARTESIAN_POINT ( 'NONE',  ( 29.50000000000000711, -9.999999999999998224, -12.50000000000000000 ) ) ;
#3122=VERTEX_POINT ( 'NONE', #202 ) ;
#3131=ORIENTED_EDGE ( 'NONE', *, *, #8107, .F. ) ;
#3146=LINE ( 'NONE', #4034, #1111 ) ;
#3158=ORIENTED_EDGE ( 'NONE', *, *, #500, .F. ) ;
#3177=EDGE_CURVE ( 'NONE', #9108, #3195, #1373, .T. ) ;
#3180=CARTESIAN_POINT ( 'NONE',  ( 34.69563600136375214, 4.609751841799207384, 2.519143709543159471 ) ) ;
#3190=DIRECTION ( 'NONE',  ( 0.000000000000000000, 0.000000000000000000, 1.000000000000000000 ) ) ;
#3195=VERTEX_POINT ( 'NONE', #4610 ) ;
#3208=ORIENTED_EDGE ( 'NONE', *, *, #1805, .F. ) ;
#3210=EDGE_LOOP ( 'NONE', ( #4076, #3440, #9214, #10338, #5343, #4622, #6043, #2586 ) ) ;
#3224=CARTESIAN_POINT ( 'NONE',  ( 34.99999999999987210, -9.999999999999998224, -10.50000000000001243 ) ) ;
#3240=FACE_BOUND ( 'NONE', #8928, .T. ) ;
#3280=DIRECTION ( 'NONE',  ( 0.000000000000000000, -0.000000000000000000, -1.000000000000000000 ) ) ;
#3281=EDGE_LOOP ( 'NONE', ( #8547, #2045, #3514, #2363 ) ) ;
#3293=DIRECTION ( 'NONE',  ( 1.000000000000000000, 0.000000000000000000, 0.000000000000000000 ) ) ;
#3294=CARTESIAN_POINT ( 'NONE',  ( -4.379688272585405606, 36.08837668307224789, -2.499999999999998668 ) ) ;
#3303=DIRECTION ( 'NONE',  ( 1.000000000000000000, 0.000000000000000000, 0.000000000000000000 ) ) ;
#3312=VERTEX_POINT ( 'NONE', #10093 ) ;
#3319=CARTESIAN_POINT ( 'NONE',  ( 29.50000000000000711, 2.000000000000001776, -10.49999999999999822 ) ) ;
#3334=DIRECTION ( 'NONE',  ( -4.312387734421975126E-17, 0.7071067811865451302, 0.7071067811865500152 ) ) ;
#3352=DIRECTION ( 'NONE',  ( -1.000000000000000000, 0.000000000000000000, 0.000000000000000000 ) ) ;
#3356=CARTESIAN_POINT ( 'NONE',  ( 25.58039891549807976, 2.000000000000002665, 2.500000000000000444 ) ) ;
#3381=VERTEX_POINT ( 'NONE', #1532 ) ;
#3383=ORIENTED_EDGE ( 'NONE', *, *, #8476, .F. ) ;
#3384=CARTESIAN_POINT ( 'NONE',  ( 25.78460820925620922, 50.00384911698630930, -2.500000000000000000 ) ) ;
#3390=DIRECTION ( 'NONE',  ( 4.312387734421982522E-17, -0.7071067811865462405, 0.7071067811865487940 ) ) ;
#3401=ORIENTED_EDGE ( 'NONE', *, *, #7038, .F. ) ;
#3408=EDGE_CURVE ( 'NONE', #10201, #1840, #8359, .T. ) ;
#3416=DIRECTION ( 'NONE',  ( 1.000000000000000000, 6.098637220230963674E-17, -0.000000000000000000 ) ) ;
#3431=DIRECTION ( 'NONE',  ( -0.000000000000000000, 0.000000000000000000, 1.000000000000000000 ) ) ;
#3440=ORIENTED_EDGE ( 'NONE', *, *, #4707, .T. ) ;
#3448=DIRECTION ( 'NONE',  ( -0.000000000000000000, -0.000000000000000000, -1.000000000000000000 ) ) ;
#3453=VECTOR ( 'NONE', #7609, 1000.000000000000000 ) ;
#3461=VECTOR ( 'NONE', #9188, 1000.000000000000000 ) ;
#3472=CARTESIAN_POINT ( 'NONE',  ( 29.50000000000000711, -9.999999999999998224, -10.50000000000001243 ) ) ;
#3477=LINE ( 'NONE', #6797, #5625 ) ;
#3483=DIRECTION ( 'NONE',  ( 0.000000000000000000, 0.000000000000000000, -1.000000000000000000 ) ) ;
#3484=LINE ( 'NONE', #4317, #10204 ) ;
#3491=AXIS2_PLACEMENT_3D ( 'NONE', #102, #5490, #1833 ) ;
#3494=VERTEX_POINT ( 'NONE', #81 ) ;
#3499=CYLINDRICAL_SURFACE ( 'NONE', #8413, 7.500000000000000000 ) ;
#3501=ORIENTED_EDGE ( 'NONE', *, *, #5607, .T. ) ;
#3504=LINE ( 'NONE', #5335, #7016 ) ;
#3513=LINE ( 'NONE', #3673, #1207 ) ;
#3514=ORIENTED_EDGE ( 'NONE', *, *, #6957, .F. ) ;
#3522=MECHANICAL_DESIGN_GEOMETRIC_PRESENTATION_REPRESENTATION('',(#4233),#4041);
#3531=EDGE_CURVE ( 'NONE', #381, #9804, #6924, .T. ) ;
#3532=VECTOR ( 'NONE', #1120, 1000.000000000000000 ) ;
#3560=EDGE_CURVE ( 'NONE', #381, #7106, #6138, .T. ) ;
#3563=EDGE_CURVE ( 'NONE', #8370, #3879, #8587, .T. ) ;
#3580=EDGE_CURVE ( 'NONE', #1107, #3494, #1815, .T. ) ;
#3583=ORIENTED_EDGE ( 'NONE', *, *, #7475, .T. ) ;
#3596=CIRCLE ( 'NONE', #558, 2.149999999999995470 ) ;
#3603=CIRCLE ( 'NONE', #4498, 4.500000000000000000 ) ;
#3621=SURFACE_STYLE_FILL_AREA ( #1909 ) ;
#3633=EDGE_CURVE ( 'NONE', #8370, #4598, #10732, .T. ) ;
#3639=AXIS2_PLACEMENT_3D ( 'NONE', #9070, #5792, #8347 ) ;
#3644=EDGE_LOOP ( 'NONE', ( #8151, #3583, #2182, #10689 ) ) ;
#3657=AXIS2_PLACEMENT_3D ( 'NONE', #1305, #2189, #10644 ) ;
#3658=ORIENTED_EDGE ( 'NONE', *, *, #9220, .T. ) ;
#3661=PLANE ( 'NONE',  #5585 ) ;
#3669=DIRECTION ( 'NONE',  ( -4.312387734421975126E-17, 0.7071067811865451302, -0.7071067811865500152 ) ) ;
#3673=CARTESIAN_POINT ( 'NONE',  ( 34.99999999999987210, -3.999999999999989786, 7.850000000000005862 ) ) ;
#3684=CARTESIAN_POINT ( 'NONE',  ( 29.50000000000000711, 2.000000000000001776, -12.50000000000000000 ) ) ;
#3696=ADVANCED_FACE ( 'NONE', ( #7980, #6244 ), #7245, .F. ) ;
#3698=DIRECTION ( 'NONE',  ( 1.000000000000000000, -0.000000000000000000, -0.000000000000000000 ) ) ;
#3701=EDGE_CURVE ( 'NONE', #6726, #2280, #459, .T. ) ;
#3741=CARTESIAN_POINT ( 'NONE',  ( 0.000000000000000000, 0.000000000000000000, 14.50000000000000000 ) ) ;
#3742=FACE_BOUND ( 'NONE', #10708, .T. ) ;
#3759=ADVANCED_FACE ( 'NONE', ( #8030, #3913 ), #10589, .F. ) ;
#3760=LINE ( 'NONE', #10487, #1327 ) ;
#3761=CARTESIAN_POINT ( 'NONE',  ( 25.98076211353311749, 56.49999999999984368, 10.00000000000000178 ) ) ;
#3782=CARTESIAN_POINT ( 'NONE',  ( 5.621179405865841083, 34.96511249490581719, -2.499999999999999112 ) ) ;
#3784=EDGE_LOOP ( 'NONE', ( #4150, #5129, #489, #832 ) ) ;
#3793=CARTESIAN_POINT ( 'NONE',  ( 34.99999999999987210, -3.999999999999989786, -7.149999999999994138 ) ) ;
#3794=ORIENTED_EDGE ( 'NONE', *, *, #5136, .T. ) ;
#3812=CIRCLE ( 'NONE', #10896, 2.149999999999992362 ) ;
#3816=CARTESIAN_POINT ( 'NONE',  ( 25.98076211353311749, 56.49999999999984368, 10.00000000000000178 ) ) ;
#3822=CIRCLE ( 'NONE', #8079, 2.149999999999995470 ) ;
#3829=VECTOR ( 'NONE', #7761, 1000.000000000000114 ) ;
#3836=ORIENTED_EDGE ( 'NONE', *, *, #9273, .F. ) ;
#3846=DIRECTION ( 'NONE',  ( 4.312387734422005941E-17, -0.7071067811865500152, 0.7071067811865451302 ) ) ;
#3861=UNCERTAINTY_MEASURE_WITH_UNIT (LENGTH_MEASURE( 1.000000000000000082E-05 ), #4997, 'distance_accuracy_value', 'NONE');
#3879=VERTEX_POINT ( 'NONE', #6679 ) ;
#3913=FACE_OUTER_BOUND ( 'NONE', #1607, .T. ) ;
#3915=CARTESIAN_POINT ( 'NONE',  ( 21.21106610644839208, 56.49999999999984368, 14.50000000000000000 ) ) ;
#3917=CARTESIAN_POINT ( 'NONE',  ( -3.049318610115481714E-16, 5.000000000000000000, -5.500000000000000000 ) ) ;
#3926=DIRECTION ( 'NONE',  ( 0.000000000000000000, 0.000000000000000000, -1.000000000000000000 ) ) ;
#3940=DIRECTION ( 'NONE',  ( 0.000000000000000000, -1.000000000000000000, 0.000000000000000000 ) ) ;
#3960=FACE_OUTER_BOUND ( 'NONE', #4066, .T. ) ;
#3963=ORIENTED_EDGE ( 'NONE', *, *, #10153, .T. ) ;
#3967=FACE_OUTER_BOUND ( 'NONE', #2410, .T. ) ;
#3984=ORIENTED_EDGE ( 'NONE', *, *, #5002, .T. ) ;
#3994=EDGE_LOOP ( 'NONE', ( #6071, #6195, #7981, #7395 ) ) ;
#4012=CARTESIAN_POINT ( 'NONE',  ( 34.66939513580730647, 4.803384628401709655, 2.499999999999999556 ) ) ;
#4018=CARTESIAN_POINT ( 'NONE',  ( 24.99999259214812142, 30.01924558493218598, 2.500000000000000000 ) ) ;
#4032=VECTOR ( 'NONE', #10535, 1000.000000000000000 ) ;
#4034=CARTESIAN_POINT ( 'NONE',  ( 29.50000000000000711, 1.387778780781445676E-14, 17.49999999999999645 ) ) ;
#4041=( GEOMETRIC_REPRESENTATION_CONTEXT ( 3 ) GLOBAL_UNCERTAINTY_ASSIGNED_CONTEXT ( ( #2529 ) ) GLOBAL_UNIT_ASSIGNED_CONTEXT ( ( #1114, #6063, #4469 ) ) REPRESENTATION_CONTEXT ( 'NONE', 'WORKASPACE' ) );
#4066=EDGE_LOOP ( 'NONE', ( #1224, #891, #8538, #592, #4500, #3107, #3501, #9461 ) ) ;
#4076=ORIENTED_EDGE ( 'NONE', *, *, #8256, .F. ) ;
#4077=DIRECTION ( 'NONE',  ( -1.000000000000000000, 0.000000000000000000, 0.000000000000000000 ) ) ;
#4082=EDGE_CURVE ( 'NONE', #3312, #1951, #8529, .T. ) ;
#4084=DIRECTION ( 'NONE',  ( -1.000000000000000000, 0.000000000000000000, 0.000000000000000000 ) ) ;
#4085=CARTESIAN_POINT ( 'NONE',  ( 34.94281041931230902, 2.000000000000002220, 5.102623512424888652 ) ) ;
#4089=ORIENTED_EDGE ( 'NONE', *, *, #7793, .T. ) ;
#4090=DIRECTION ( 'NONE',  ( -1.000000000000000000, -6.098637220230963674E-17, 0.000000000000000000 ) ) ;
#4102=CARTESIAN_POINT ( 'NONE',  ( 29.50000000000000711, 2.000000000000001776, 17.49999999999999645 ) ) ;
#4104=ORIENTED_EDGE ( 'NONE', *, *, #10897, .T. ) ;
#4129=ORIENTED_EDGE ( 'NONE', *, *, #5268, .T. ) ;
#4136=CARTESIAN_POINT ( 'NONE',  ( 29.17190429162964094, 2.000000000000001776, 2.500000000000000444 ) ) ;
#4149=DIRECTION ( 'NONE',  ( 1.000000000000000000, -8.673617379884033500E-16, 0.000000000000000000 ) ) ;
#4150=ORIENTED_EDGE ( 'NONE', *, *, #6607, .T. ) ;
#4160=LINE ( 'NONE', #7556, #8073 ) ;
#4162=DIRECTION ( 'NONE',  ( -0.000000000000000000, 0.000000000000000000, 1.000000000000000000 ) ) ;
#4165=CARTESIAN_POINT ( 'NONE',  ( 29.17190429162964094, 7.000000000000002665, 2.500000000000000000 ) ) ;
#4166=ADVANCED_FACE ( 'NONE', ( #9294 ), #852, .F. ) ;
#4183=DIRECTION ( 'NONE',  ( -0.000000000000000000, -0.000000000000000000, -1.000000000000000000 ) ) ;
#4184=AXIS2_PLACEMENT_3D ( 'NONE', #1253, #9803, #5423 ) ;
#4194=AXIS2_PLACEMENT_3D ( 'NONE', #3741, #6187, #8694 ) ;
#4207=DIRECTION ( 'NONE',  ( -1.000000000000000000, -6.098637220230963674E-17, 0.000000000000000000 ) ) ;
#4210=CARTESIAN_POINT ( 'NONE',  ( 25.98076211353324183, 54.99999999999984368, 2.500000000000000000 ) ) ;
#4225=EDGE_CURVE ( 'NONE', #6073, #6168, #10927, .T. ) ;
#4230=DIRECTION ( 'NONE',  ( 0.000000000000000000, 0.000000000000000000, 1.000000000000000000 ) ) ;
#4233=STYLED_ITEM ( 'NONE', ( #176 ), #2840 ) ;
#4237=ORIENTED_EDGE ( 'NONE', *, *, #8319, .F. ) ;
#4238=VECTOR ( 'NONE', #7135, 1000.000000000000000 ) ;
#4241=EDGE_CURVE ( 'NONE', #8894, #3195, #9357, .T. ) ;
#4249=CARTESIAN_POINT ( 'NONE',  ( 34.99999999999987210, -17.99999999999996803, 7.500000000000038192 ) ) ;
#4259=DIRECTION ( 'NONE',  ( 1.000000000000000000, 0.000000000000000000, 0.000000000000000000 ) ) ;
#4264=ORIENTED_EDGE ( 'NONE', *, *, #10502, .T. ) ;
#4270=CARTESIAN_POINT ( 'NONE',  ( 25.58039891549807976, 2.000000000000002665, 17.50099999999999767 ) ) ;
#4291=LINE ( 'NONE', #7679, #5473 ) ;
#4296=DIRECTION ( 'NONE',  ( 0.000000000000000000, 0.000000000000000000, 1.000000000000000000 ) ) ;
#4316=FACE_OUTER_BOUND ( 'NONE', #10872, .T. ) ;
#4317=CARTESIAN_POINT ( 'NONE',  ( 5.621179405865834866, 34.96511249490581008, 0.000000000000000000 ) ) ;
#4319=ORIENTED_EDGE ( 'NONE', *, *, #9220, .F. ) ;
#4321=DIRECTION ( 'NONE',  ( 0.000000000000000000, 0.000000000000000000, 1.000000000000000000 ) ) ;
#4328=ORIENTED_EDGE ( 'NONE', *, *, #7475, .F. ) ;
#4333=SHAPE_DEFINITION_REPRESENTATION ( #2103, #3016 ) ;
#4342=EDGE_CURVE ( 'NONE', #1437, #40, #1016, .T. ) ;
#4343=DIRECTION ( 'NONE',  ( -1.000000000000000000, 0.000000000000000000, 0.000000000000000000 ) ) ;
#4357=AXIS2_PLACEMENT_3D ( 'NONE', #4210, #2774, #6146 ) ;
#4362=PLANE ( 'NONE',  #5984 ) ;
#4364=ORIENTED_EDGE ( 'NONE', *, *, #3580, .T. ) ;
#4378=CARTESIAN_POINT ( 'NONE',  ( 24.99999259214812142, 30.01924558493218598, -2.500000000000000000 ) ) ;
#4386=ADVANCED_FACE ( 'NONE', ( #1973 ), #1919, .F. ) ;
#4390=ORIENTED_EDGE ( 'NONE', *, *, #7287, .F. ) ;
#4407=CARTESIAN_POINT ( 'NONE',  ( 25.71106610644839208, 56.49999999999984368, 10.00000000000000178 ) ) ;
#4417=CARTESIAN_POINT ( 'NONE',  ( 25.98076211353311749, 53.49999999999983658, 7.850000000000012967 ) ) ;
#4427=ORIENTED_EDGE ( 'NONE', *, *, #10502, .F. ) ;
#4431=AXIS2_PLACEMENT_3D ( 'NONE', #4165, #7559, #8135 ) ;
#4432=CARTESIAN_POINT ( 'NONE',  ( -2.649999999999885780, 30.00000000000000000, 2.500000000000000000 ) ) ;
#4455=DIRECTION ( 'NONE',  ( 1.000000000000000000, 6.098637220230963674E-17, 0.000000000000000000 ) ) ;
#4459=DIRECTION ( 'NONE',  ( 0.000000000000000000, 1.000000000000000000, 0.000000000000000000 ) ) ;
#4464=LINE ( 'NONE', #6169, #8658 ) ;
#4467=ORIENTED_EDGE ( 'NONE', *, *, #498, .T. ) ;
#4469=( NAMED_UNIT ( * ) SI_UNIT ( $, .STERADIAN. ) SOLID_ANGLE_UNIT ( ) );
#4486=CARTESIAN_POINT ( 'NONE',  ( 25.98076211353311749, 56.49999999999984368, 7.850000000000012967 ) ) ;
#4489=ADVANCED_FACE ( 'NONE', ( #934 ), #2098, .F. ) ;
#4498=AXIS2_PLACEMENT_3D ( 'NONE', #4407, #8098, #3926 ) ;
#4500=ORIENTED_EDGE ( 'NONE', *, *, #2218, .T. ) ;
#4517=EDGE_CURVE ( 'NONE', #681, #9108, #8090, .T. ) ;
#4518=FACE_OUTER_BOUND ( 'NONE', #10135, .T. ) ;
#4519=ADVANCED_FACE ( 'NONE', ( #4813 ), #1309, .F. ) ;
#4524=CYLINDRICAL_SURFACE ( 'NONE', #7223, 4.500000000000000888 ) ;
#4533=DIRECTION ( 'NONE',  ( 0.000000000000000000, -0.000000000000000000, -1.000000000000000000 ) ) ;
#4534=AXIS2_PLACEMENT_3D ( 'NONE', #5281, #3390, #4455 ) ;
#4544=CYLINDRICAL_SURFACE ( 'NONE', #2825, 3.000000000000000000 ) ;
#4552=CARTESIAN_POINT ( 'NONE',  ( 34.99999999999987210, -3.999999999999989786, 9.999999999999998224 ) ) ;
#4564=ORIENTED_EDGE ( 'NONE', *, *, #8797, .T. ) ;
#4567=DIRECTION ( 'NONE',  ( 0.000000000000000000, 0.000000000000000000, 1.000000000000000000 ) ) ;
#4570=ORIENTED_EDGE ( 'NONE', *, *, #6544, .F. ) ;
#4579=AXIS2_PLACEMENT_3D ( 'NONE', #284, #10401, #8627 ) ;
#4586=DIRECTION ( 'NONE',  ( -1.000000000000000000, -6.098637220230963674E-17, 0.000000000000000000 ) ) ;
#4592=CARTESIAN_POINT ( 'NONE',  ( 21.21106610644839208, 53.49999999999983658, 10.00000000000000178 ) ) ;
#4597=EDGE_CURVE ( 'NONE', #3494, #7883, #1471, .T. ) ;
#4598=VERTEX_POINT ( 'NONE', #10694 ) ;
#4606=DIRECTION ( 'NONE',  ( 0.000000000000000000, 0.000000000000000000, 1.000000000000000000 ) ) ;
#4610=CARTESIAN_POINT ( 'NONE',  ( 30.75045812061784289, 53.49999999999983658, 2.500000000000000000 ) ) ;
#4612=EDGE_LOOP ( 'NONE', ( #5221, #379, #5238, #1445 ) ) ;
#4620=ORIENTED_EDGE ( 'NONE', *, *, #8319, .T. ) ;
#4622=ORIENTED_EDGE ( 'NONE', *, *, #1402, .T. ) ;
#4630=DIRECTION ( 'NONE',  ( 1.000000000000000000, 0.000000000000000000, 0.000000000000000000 ) ) ;
#4633=DIRECTION ( 'NONE',  ( -0.000000000000000000, -0.000000000000000000, -1.000000000000000000 ) ) ;
#4638=DIRECTION ( 'NONE',  ( -0.000000000000000000, 0.000000000000000000, 1.000000000000000000 ) ) ;
#4653=DIRECTION ( 'NONE',  ( -6.098637220230963674E-17, 1.000000000000000000, 0.000000000000000000 ) ) ;
#4654=ADVANCED_FACE ( 'NONE', ( #629 ), #5590, .T. ) ;
#4675=DIRECTION ( 'NONE',  ( 1.000000000000000000, 0.000000000000000000, 0.000000000000000000 ) ) ;
#4676=ORIENTED_EDGE ( 'NONE', *, *, #7169, .T. ) ;
#4684=DIRECTION ( 'NONE',  ( 0.000000000000000000, 0.000000000000000000, -1.000000000000000000 ) ) ;
#4702=ORIENTED_EDGE ( 'NONE', *, *, #7653, .F. ) ;
#4707=EDGE_CURVE ( 'NONE', #10104, #7106, #3477, .T. ) ;
#4710=FACE_OUTER_BOUND ( 'NONE', #10933, .T. ) ;
#4729=VERTEX_POINT ( 'NONE', #7754 ) ;
#4745=VECTOR ( 'NONE', #4863, 1000.000000000000000 ) ;
#4752=DIRECTION ( 'NONE',  ( -0.000000000000000000, 1.000000000000000000, -0.000000000000000000 ) ) ;
#4766=CARTESIAN_POINT ( 'NONE',  ( 5.076455387921338769, 24.47916666666667140, 0.000000000000000000 ) ) ;
#4784=EDGE_LOOP ( 'NONE', ( #6994, #5194 ) ) ;
#4797=DIRECTION ( 'NONE',  ( 0.000000000000000000, 0.000000000000000000, -1.000000000000000000 ) ) ;
#4800=ORIENTED_EDGE ( 'NONE', *, *, #4342, .F. ) ;
#4804=DIRECTION ( 'NONE',  ( 0.000000000000000000, -0.000000000000000000, -1.000000000000000000 ) ) ;
#4806=FACE_OUTER_BOUND ( 'NONE', #5220, .T. ) ;
#4808=DIRECTION ( 'NONE',  ( 1.000000000000000000, 0.000000000000000000, 0.000000000000000000 ) ) ;
#4813=FACE_OUTER_BOUND ( 'NONE', #3281, .T. ) ;
#4819=EDGE_CURVE ( 'NONE', #9208, #874, #5309, .T. ) ;
#4837=DIRECTION ( 'NONE',  ( 1.000000000000000000, 0.000000000000000000, 0.000000000000000000 ) ) ;
#4845=CARTESIAN_POINT ( 'NONE',  ( 34.93373351399774407, 2.154066368359273564, -4.530732988813361395 ) ) ;
#4849=VERTEX_POINT ( 'NONE', #8695 ) ;
#4863=DIRECTION ( 'NONE',  ( 1.000000000000000000, 6.098637220230963674E-17, 0.000000000000000000 ) ) ;
#4866=ADVANCED_FACE ( 'NONE', ( #3742, #2865 ), #295, .T. ) ;
#4868=CARTESIAN_POINT ( 'NONE',  ( 34.91780110604603493, 2.399866884679865198, 3.990594396599065341 ) ) ;
#4905=CARTESIAN_POINT ( 'NONE',  ( 34.64101615137754919, 5.000000000000002665, -2.500000000000000000 ) ) ;
#4913=CARTESIAN_POINT ( 'NONE',  ( 6.015568632492061418, 34.47916666666664298, 2.500000000000000000 ) ) ;
#4914=DIRECTION ( 'NONE',  ( 0.000000000000000000, -0.000000000000000000, -1.000000000000000000 ) ) ;
#4932=ADVANCED_FACE ( 'NONE', ( #9744 ), #1298, .F. ) ;
#4953=STYLED_ITEM ( 'NONE', ( #6086 ), #5541 ) ;
#4978=DIRECTION ( 'NONE',  ( 1.000000000000000000, -0.000000000000000000, -0.000000000000000000 ) ) ;
#4982=CARTESIAN_POINT ( 'NONE',  ( 34.82458596820517016, 3.503579405888651799, 2.892497030208067699 ) ) ;
#4986=ORIENTED_EDGE ( 'NONE', *, *, #1832, .T. ) ;
#4997=( LENGTH_UNIT ( ) NAMED_UNIT ( * ) SI_UNIT ( .MILLI., .METRE. ) );
#5000=LINE ( 'NONE', #8375, #3453 ) ;
#5002=EDGE_CURVE ( 'NONE', #6726, #10201, #2770, .T. ) ;
#5007=CARTESIAN_POINT ( 'NONE',  ( 25.98076211353324183, 54.99999999999984368, 2.500000000000000000 ) ) ;
#5015=LINE ( 'NONE', #8391, #1384 ) ;
#5017=ORIENTED_EDGE ( 'NONE', *, *, #305, .F. ) ;
#5022=ADVANCED_FACE ( 'NONE', ( #10151, #7478, #8363 ), #7596, .T. ) ;
#5030=ORIENTED_EDGE ( 'NONE', *, *, #953, .F. ) ;
#5039=CARTESIAN_POINT ( 'NONE',  ( 26.17691601781025312, 59.99615088301337096, 2.500000000000000000 ) ) ;
#5054=VERTEX_POINT ( 'NONE', #918 ) ;
#5061=DIRECTION ( 'NONE',  ( 0.000000000000000000, -1.000000000000000000, 0.000000000000000000 ) ) ;
#5064=VECTOR ( 'NONE', #3448, 1000.000000000000000 ) ;
#5067=EDGE_CURVE ( 'NONE', #3195, #3312, #6522, .T. ) ;
#5107=LINE ( 'NONE', #7659, #926 ) ;
#5108=VECTOR ( 'NONE', #405, 1000.000000000000000 ) ;
#5114=EDGE_LOOP ( 'NONE', ( #2497, #10874, #10577, #322, #1281, #9847 ) ) ;
#5129=ORIENTED_EDGE ( 'NONE', *, *, #6338, .T. ) ;
#5130=DIRECTION ( 'NONE',  ( -0.000000000000000000, -0.000000000000000000, -1.000000000000000000 ) ) ;
#5134=EDGE_LOOP ( 'NONE', ( #10655, #5180, #1337, #542 ) ) ;
#5136=EDGE_CURVE ( 'NONE', #8126, #1456, #1592, .T. ) ;
#5146=EDGE_LOOP ( 'NONE', ( #5443, #3383 ) ) ;
#5147=DIRECTION ( 'NONE',  ( 0.000000000000000000, 0.000000000000000000, -1.000000000000000000 ) ) ;
#5155=CARTESIAN_POINT ( 'NONE',  ( 0.000000000000000000, 30.00000000000000000, 2.500000000000000000 ) ) ;
#5180=ORIENTED_EDGE ( 'NONE', *, *, #10764, .T. ) ;
#5184=ORIENTED_EDGE ( 'NONE', *, *, #10658, .F. ) ;
#5192=DIRECTION ( 'NONE',  ( 0.000000000000000000, -0.000000000000000000, 1.000000000000000000 ) ) ;
#5193=ADVANCED_FACE ( 'NONE', ( #6088 ), #4544, .F. ) ;
#5194=ORIENTED_EDGE ( 'NONE', *, *, #3633, .F. ) ;
#5195=ORIENTED_EDGE ( 'NONE', *, *, #6672, .F. ) ;
#5218=DIRECTION ( 'NONE',  ( 4.312387734421975126E-17, -0.7071067811865451302, 0.7071067811865500152 ) ) ;
#5220=EDGE_LOOP ( 'NONE', ( #5195, #1766, #6385, #9462 ) ) ;
#5221=ORIENTED_EDGE ( 'NONE', *, *, #867, .F. ) ;
#5222=DIRECTION ( 'NONE',  ( 1.000000000000000000, 6.098637220230963674E-17, -0.000000000000000000 ) ) ;
#5227=CARTESIAN_POINT ( 'NONE',  ( 1.047444401652940007E-13, 30.00000000000000000, -2.500000000000000000 ) ) ;
#5234=DIRECTION ( 'NONE',  ( 1.000000000000000000, -0.000000000000000000, -0.000000000000000000 ) ) ;
#5238=ORIENTED_EDGE ( 'NONE', *, *, #302, .F. ) ;
#5240=CIRCLE ( 'NONE', #2935, 7.500000000000000000 ) ;
#5250=ORIENTED_EDGE ( 'NONE', *, *, #5677, .T. ) ;
#5268=EDGE_CURVE ( 'NONE', #2494, #1437, #6961, .T. ) ;
#5272=AXIS2_PLACEMENT_3D ( 'NONE', #5525, #8907, #8023 ) ;
#5281=CARTESIAN_POINT ( 'NONE',  ( 6.098637220230963427E-16, -10.00000000000000000, 15.49999999999998934 ) ) ;
#5282=LINE ( 'NONE', #8719, #2588 ) ;
#5290=PRODUCT ( 'caliper arm left', 'caliper arm left', '', ( #1044 ) ) ;
#5291=ORIENTED_EDGE ( 'NONE', *, *, #5967, .T. ) ;
#5292=VECTOR ( 'NONE', #10723, 1000.000000000000000 ) ;
#5297=SURFACE_SIDE_STYLE ('',( #3621 ) ) ;
#5300=( GEOMETRIC_REPRESENTATION_CONTEXT ( 3 ) GLOBAL_UNCERTAINTY_ASSIGNED_CONTEXT ( ( #3861 ) ) GLOBAL_UNIT_ASSIGNED_CONTEXT ( ( #4997, #6980, #1869 ) ) REPRESENTATION_CONTEXT ( 'NONE', 'WORKASPACE' ) );
#5309=LINE ( 'NONE', #6917, #9158 ) ;
#5310=VECTOR ( 'NONE', #8287, 1000.000000000000000 ) ;
#5316=DIRECTION ( 'NONE',  ( 0.000000000000000000, 0.000000000000000000, 1.000000000000000000 ) ) ;
#5317=CARTESIAN_POINT ( 'NONE',  ( 29.50000000000000711, 2.000000000000001776, 5.500000000000000000 ) ) ;
#5319=SURFACE_STYLE_FILL_AREA ( #972 ) ;
#5323=DIRECTION ( 'NONE',  ( 1.000000000000000000, -0.000000000000000000, -0.000000000000000000 ) ) ;
#5329=CARTESIAN_POINT ( 'NONE',  ( 25.78460820925620922, 50.00384911698630930, 2.500000000000000000 ) ) ;
#5332=ORIENTED_EDGE ( 'NONE', *, *, #6636, .T. ) ;
#5334=CARTESIAN_POINT ( 'NONE',  ( 34.99999999999987210, -3.999999999999989786, 9.999999999999998224 ) ) ;
#5335=CARTESIAN_POINT ( 'NONE',  ( 25.98076211353311749, 56.49999999999984368, 12.14999999999999147 ) ) ;
#5343=ORIENTED_EDGE ( 'NONE', *, *, #6530, .F. ) ;
#5387=EDGE_CURVE ( 'NONE', #7883, #3122, #8901, .T. ) ;
#5390=EDGE_CURVE ( 'NONE', #3024, #6057, #7018, .T. ) ;
#5394=CARTESIAN_POINT ( 'NONE',  ( 29.50000000000000711, 2.000000000000001776, 15.49999999999999645 ) ) ;
#5407=CARTESIAN_POINT ( 'NONE',  ( 26.25045812061784289, 56.49999999999984368, 10.00000000000000178 ) ) ;
#5423=DIRECTION ( 'NONE',  ( 0.000000000000000000, -1.000000000000000000, 0.000000000000000000 ) ) ;
#5440=LINE ( 'NONE', #1094, #1314 ) ;
#5443=ORIENTED_EDGE ( 'NONE', *, *, #1449, .F. ) ;
#5448=ORIENTED_EDGE ( 'NONE', *, *, #7524, .T. ) ;
#5462=AXIS2_PLACEMENT_3D ( 'NONE', #7693, #10132, #127 ) ;
#5463=AXIS2_PLACEMENT_3D ( 'NONE', #5516, #6439, #4684 ) ;
#5468=ORIENTED_EDGE ( 'NONE', *, *, #4517, .T. ) ;
#5473=VECTOR ( 'NONE', #5234, 1000.000000000000000 ) ;
#5490=DIRECTION ( 'NONE',  ( 1.000000000000000000, 0.000000000000000000, 0.000000000000000000 ) ) ;
#5496=DIRECTION ( 'NONE',  ( 1.000000000000000000, 6.098637220230963674E-17, 0.000000000000000000 ) ) ;
#5503=DIRECTION ( 'NONE',  ( 0.000000000000000000, 0.000000000000000000, 1.000000000000000000 ) ) ;
#5506=ORIENTED_EDGE ( 'NONE', *, *, #305, .T. ) ;
#5509=CARTESIAN_POINT ( 'NONE',  ( 1.047444401652940007E-13, 30.00000000000000000, 2.500000000000000000 ) ) ;
#5516=CARTESIAN_POINT ( 'NONE',  ( 34.99999999999987210, -3.999999999999989786, -4.999999999999999112 ) ) ;
#5525=CARTESIAN_POINT ( 'NONE',  ( 1.047444401652940007E-13, 30.00000000000000000, -2.500000000000000000 ) ) ;
#5527=CIRCLE ( 'NONE', #373, 7.500000000000000000 ) ;
#5541=MANIFOLD_SOLID_BREP ( 'Fillet4', #10725 ) ;
#5542=EDGE_CURVE ( 'NONE', #6762, #7090, #1933, .T. ) ;
#5548=AXIS2_PLACEMENT_3D ( 'NONE', #4270, #1037, #8487 ) ;
#5573=CARTESIAN_POINT ( 'NONE',  ( 34.92408131826248052, 2.305272916965853014, -4.166859826334558647 ) ) ;
#5585=AXIS2_PLACEMENT_3D ( 'NONE', #7054, #2839, #6211 ) ;
#5590=PLANE ( 'NONE',  #7019 ) ;
#5601=AXIS2_PLACEMENT_3D ( 'NONE', #3917, #7354, #8192 ) ;
#5602=VECTOR ( 'NONE', #10876, 1000.000000000000000 ) ;
#5607=EDGE_CURVE ( 'NONE', #8525, #7309, #2930, .T. ) ;
#5611=VECTOR ( 'NONE', #9082, 1000.000000000000000 ) ;
#5623=DIRECTION ( 'NONE',  ( 1.000000000000000000, 6.098637220230963674E-17, -0.000000000000000000 ) ) ;
#5625=VECTOR ( 'NONE', #3416, 1000.000000000000000 ) ;
#5636=AXIS2_PLACEMENT_3D ( 'NONE', #2332, #7442, #8275 ) ;
#5645=VECTOR ( 'NONE', #3069, 1000.000000000000000 ) ;
#5656=ORIENTED_EDGE ( 'NONE', *, *, #5390, .F. ) ;
#5677=EDGE_CURVE ( 'NONE', #10983, #1951, #1307, .T. ) ;
#5680=DIRECTION ( 'NONE',  ( 0.000000000000000000, 0.000000000000000000, -1.000000000000000000 ) ) ;
#5681=ORIENTED_EDGE ( 'NONE', *, *, #8372, .T. ) ;
#5683=ORIENTED_EDGE ( 'NONE', *, *, #460, .T. ) ;
#5697=DIRECTION ( 'NONE',  ( -1.000000000000000000, 0.000000000000000000, 0.000000000000000000 ) ) ;
#5704=ORIENTED_EDGE ( 'NONE', *, *, #3633, .T. ) ;
#5746=CYLINDRICAL_SURFACE ( 'NONE', #9659, 34.99999999999999289 ) ;
#5763=AXIS2_PLACEMENT_3D ( 'NONE', #371, #1098, #5503 ) ;
#5780=CARTESIAN_POINT ( 'NONE',  ( 34.74482695545610511, 4.223122737142881888, -2.595677240809973085 ) ) ;
#5792=DIRECTION ( 'NONE',  ( 1.000000000000000000, 6.098637220230963674E-17, -0.000000000000000000 ) ) ;
#5793=DIRECTION ( 'NONE',  ( -0.000000000000000000, -0.000000000000000000, -1.000000000000000000 ) ) ;
#5806=CARTESIAN_POINT ( 'NONE',  ( 29.50000000000000711, -7.999999999999983125, 17.49999999999999645 ) ) ;
#5813=DIRECTION ( 'NONE',  ( -1.000000000000000000, -6.098637220230963674E-17, 0.000000000000000000 ) ) ;
#5823=ORIENTED_EDGE ( 'NONE', *, *, #6672, .T. ) ;
#5826=ADVANCED_FACE ( 'NONE', ( #10738 ), #7577, .F. ) ;
#5832=CIRCLE ( 'NONE', #8681, 4.500000000000000888 ) ;
#5839=LINE ( 'NONE', #112, #788 ) ;
#5840=ORIENTED_EDGE ( 'NONE', *, *, #5067, .F. ) ;
#5883=VECTOR ( 'NONE', #7715, 1000.000000000000000 ) ;
#5917=CYLINDRICAL_SURFACE ( 'NONE', #6526, 4.500000000000000000 ) ;
#5921=DIRECTION ( 'NONE',  ( 6.098637220230963674E-17, -1.000000000000000000, 0.000000000000000000 ) ) ;
#5923=VECTOR ( 'NONE', #10703, 1000.000000000000114 ) ;
#5929=ORIENTED_EDGE ( 'NONE', *, *, #1202, .T. ) ;
#5930=VECTOR ( 'NONE', #6096, 1000.000000000000000 ) ;
#5935=CARTESIAN_POINT ( 'NONE',  ( 0.000000000000000000, 30.00000000000000000, -23.71320343559643007 ) ) ;
#5947=CIRCLE ( 'NONE', #4357, 4.999999999999997335 ) ;
#5967=EDGE_CURVE ( 'NONE', #9110, #183, #1376, .T. ) ;
#5984=AXIS2_PLACEMENT_3D ( 'NONE', #10300, #1852, #5192 ) ;
#6007=DIRECTION ( 'NONE',  ( -6.098637220230963674E-17, 1.000000000000000000, 0.000000000000000000 ) ) ;
#6009=AXIS2_PLACEMENT_3D ( 'NONE', #3030, #4230, #8184 ) ;
#6013=( LENGTH_UNIT ( ) NAMED_UNIT ( * ) SI_UNIT ( .MILLI., .METRE. ) );
#6014=ADVANCED_FACE ( 'NONE', ( #6020, #8690 ), #4362, .F. ) ;
#6020=FACE_BOUND ( 'NONE', #10614, .T. ) ;
#6022=VERTEX_POINT ( 'NONE', #9405 ) ;
#6043=ORIENTED_EDGE ( 'NONE', *, *, #2218, .F. ) ;
#6053=LINE ( 'NONE', #9441, #7484 ) ;
#6056=DIRECTION ( 'NONE',  ( -0.000000000000000000, -0.000000000000000000, -1.000000000000000000 ) ) ;
#6057=VERTEX_POINT ( 'NONE', #3472 ) ;
#6058=CARTESIAN_POINT ( 'NONE',  ( 24.30992024302469900, 5.833333333333334814, -2.500000000000000000 ) ) ;
#6063=( NAMED_UNIT ( * ) PLANE_ANGLE_UNIT ( ) SI_UNIT ( $, .RADIAN. ) );
#6064=CARTESIAN_POINT ( 'NONE',  ( 29.17190429162964094, 7.000000000000002665, 2.500000000000000000 ) ) ;
#6071=ORIENTED_EDGE ( 'NONE', *, *, #2056, .F. ) ;
#6073=VERTEX_POINT ( 'NONE', #3793 ) ;
#6074=ADVANCED_FACE ( 'NONE', ( #7915 ), #4524, .T. ) ;
#6078=AXIS2_PLACEMENT_3D ( 'NONE', #2789, #4459, #7840 ) ;
#6085=ORIENTED_EDGE ( 'NONE', *, *, #8721, .F. ) ;
#6086=PRESENTATION_STYLE_ASSIGNMENT (( #10367 ) ) ;
#6088=FACE_OUTER_BOUND ( 'NONE', #265, .T. ) ;
#6095=CARTESIAN_POINT ( 'NONE',  ( 34.99999999999987210, -7.999999999999983125, 17.49999999999999645 ) ) ;
#6096=DIRECTION ( 'NONE',  ( 6.098637220230963674E-17, -1.000000000000000000, 0.000000000000000000 ) ) ;
#6120=VECTOR ( 'NONE', #4633, 1000.000000000000000 ) ;
#6138=LINE ( 'NONE', #1132, #2778 ) ;
#6141=ADVANCED_FACE ( 'NONE', ( #10575 ), #2018, .F. ) ;
#6146=DIRECTION ( 'NONE',  ( 1.000000000000000000, 0.000000000000000000, 0.000000000000000000 ) ) ;
#6149=DIRECTION ( 'NONE',  ( -1.000000000000000000, -6.098637220230963674E-17, 0.000000000000000000 ) ) ;
#6151=ORIENTED_EDGE ( 'NONE', *, *, #7653, .T. ) ;
#6168=VERTEX_POINT ( 'NONE', #6184 ) ;
#6169=CARTESIAN_POINT ( 'NONE',  ( 6.015568632492064083, 34.47916666666664298, 0.000000000000000000 ) ) ;
#6174=ORIENTED_EDGE ( 'NONE', *, *, #7713, .T. ) ;
#6176=SHAPE_REPRESENTATION_RELATIONSHIP ( 'NONE' , 'NONE' ,  #3016, #2840 ) ;
#6180=CARTESIAN_POINT ( 'NONE',  ( 29.50000000000000711, 1.387778780781445676E-14, 17.49999999999999645 ) ) ;
#6184=CARTESIAN_POINT ( 'NONE',  ( 34.99999999999987210, -3.999999999999989786, -2.850000000000004530 ) ) ;
#6187=DIRECTION ( 'NONE',  ( 0.000000000000000000, 0.000000000000000000, -1.000000000000000000 ) ) ;
#6195=ORIENTED_EDGE ( 'NONE', *, *, #8047, .T. ) ;
#6201=CARTESIAN_POINT ( 'NONE',  ( 3.469446951953614189E-15, -1.040834085586084257E-14, 2.500000000000000000 ) ) ;
#6208=ORIENTED_EDGE ( 'NONE', *, *, #905, .T. ) ;
#6211=DIRECTION ( 'NONE',  ( -1.000000000000000000, -6.098637220230963674E-17, 0.000000000000000000 ) ) ;
#6227=DIRECTION ( 'NONE',  ( 0.000000000000000000, -0.000000000000000000, -1.000000000000000000 ) ) ;
#6232=DIRECTION ( 'NONE',  ( 6.098637220230963674E-17, -1.000000000000000000, 0.000000000000000000 ) ) ;
#6234=DIRECTION ( 'NONE',  ( 0.000000000000000000, 0.000000000000000000, 1.000000000000000000 ) ) ;
#6244=FACE_OUTER_BOUND ( 'NONE', #5114, .T. ) ;
#6251=CYLINDRICAL_SURFACE ( 'NONE', #9118, 2.149999999999992362 ) ;
#6263=CARTESIAN_POINT ( 'NONE',  ( 29.50000000000000711, -3.999999999999989786, 12.14999999999999147 ) ) ;
#6271=LINE ( 'NONE', #10457, #7230 ) ;
#6277=CIRCLE ( 'NONE', #8940, 3.000000000000000000 ) ;
#6293=CARTESIAN_POINT ( 'NONE',  ( 29.50000000000000711, 2.000000000000001776, -5.500000000000000000 ) ) ;
#6297=AXIS2_PLACEMENT_3D ( 'NONE', #8498, #935, #7670 ) ;
#6309=VECTOR ( 'NONE', #738, 1000.000000000000000 ) ;
#6327=EDGE_LOOP ( 'NONE', ( #3208, #6629, #3658, #5291 ) ) ;
#6329=ORIENTED_EDGE ( 'NONE', *, *, #90, .F. ) ;
#6338=EDGE_CURVE ( 'NONE', #7545, #7348, #2456, .T. ) ;
#6350=ADVANCED_FACE ( 'NONE', ( #8334 ), #6498, .F. ) ;
#6352=VECTOR ( 'NONE', #1108, 1000.000000000000000 ) ;
#6360=EDGE_CURVE ( 'NONE', #6057, #8126, #607, .T. ) ;
#6371=DIRECTION ( 'NONE',  ( -1.000000000000000000, -6.098637220230963674E-17, 0.000000000000000000 ) ) ;
#6385=ORIENTED_EDGE ( 'NONE', *, *, #8047, .F. ) ;
#6422=AXIS2_PLACEMENT_3D ( 'NONE', #2624, #6945, #4343 ) ;
#6423=CARTESIAN_POINT ( 'NONE',  ( 34.99999999999987210, -7.999999999999983125, 17.49999999999999645 ) ) ;
#6429=VERTEX_POINT ( 'NONE', #6058 ) ;
#6439=DIRECTION ( 'NONE',  ( 1.000000000000000000, -0.000000000000000000, -0.000000000000000000 ) ) ;
#6450=ADVANCED_FACE ( 'NONE', ( #1841 ), #9340, .F. ) ;
#6457=ORIENTED_EDGE ( 'NONE', *, *, #5607, .F. ) ;
#6466=EDGE_CURVE ( 'NONE', #2261, #6168, #4291, .T. ) ;
#6476=LINE ( 'NONE', #8044, #5923 ) ;
#6498=CYLINDRICAL_SURFACE ( 'NONE', #2988, 2.149999999999992362 ) ;
#6519=CARTESIAN_POINT ( 'NONE',  ( 34.99999999999987210, -3.999999999999989786, 9.999999999999998224 ) ) ;
#6522=CIRCLE ( 'NONE', #3003, 4.999999999999997335 ) ;
#6526=AXIS2_PLACEMENT_3D ( 'NONE', #9301, #79, #3483 ) ;
#6530=EDGE_CURVE ( 'NONE', #6697, #9804, #5015, .T. ) ;
#6544=EDGE_CURVE ( 'NONE', #4598, #7957, #3513, .T. ) ;
#6551=FACE_OUTER_BOUND ( 'NONE', #10396, .T. ) ;
#6554=CARTESIAN_POINT ( 'NONE',  ( 34.85635190221861279, 3.172051726186626563, -3.113055717248543797 ) ) ;
#6561=CARTESIAN_POINT ( 'NONE',  ( 1.047444401652940007E-13, 30.00000000000000000, -2.500000000000000000 ) ) ;
#6594=CIRCLE ( 'NONE', #3063, 2.149999999999994582 ) ;
#6595=CARTESIAN_POINT ( 'NONE',  ( 25.98076211353311749, 56.49999999999984368, 12.14999999999999503 ) ) ;
#6596=EDGE_CURVE ( 'NONE', #1634, #8162, #277, .T. ) ;
#6607=EDGE_CURVE ( 'NONE', #8989, #7545, #7407, .T. ) ;
#6619=DIRECTION ( 'NONE',  ( -1.000000000000000000, -0.000000000000000000, -0.000000000000000000 ) ) ;
#6621=DIRECTION ( 'NONE',  ( -0.000000000000000000, -0.000000000000000000, -1.000000000000000000 ) ) ;
#6629=ORIENTED_EDGE ( 'NONE', *, *, #905, .F. ) ;
#6631=AXIS2_PLACEMENT_3D ( 'NONE', #2829, #4653, #6371 ) ;
#6636=EDGE_CURVE ( 'NONE', #4849, #6073, #6271, .T. ) ;
#6651=AXIS2_PLACEMENT_3D ( 'NONE', #7357, #4084, #3190 ) ;
#6672=EDGE_CURVE ( 'NONE', #2549, #10302, #4464, .T. ) ;
#6679=CARTESIAN_POINT ( 'NONE',  ( 34.99999999999987210, -3.999999999999989786, 12.14999999999999503 ) ) ;
#6682=ORIENTED_EDGE ( 'NONE', *, *, #9409, .T. ) ;
#6697=VERTEX_POINT ( 'NONE', #5394 ) ;
#6699=CIRCLE ( 'NONE', #8659, 4.999999999999997335 ) ;
#6708=ORIENTED_EDGE ( 'NONE', *, *, #10435, .T. ) ;
#6710=EDGE_CURVE ( 'NONE', #3494, #3024, #217, .T. ) ;
#6717=ORIENTED_EDGE ( 'NONE', *, *, #3563, .F. ) ;
#6721=CARTESIAN_POINT ( 'NONE',  ( 29.50000000000000711, -9.999999999999998224, 15.49999999999998934 ) ) ;
#6726=VERTEX_POINT ( 'NONE', #7219 ) ;
#6733=LINE ( 'NONE', #7400, #5310 ) ;
#6749=CARTESIAN_POINT ( 'NONE',  ( 26.25045812061784289, 53.49999999999983658, 14.50000000000000000 ) ) ;
#6762=VERTEX_POINT ( 'NONE', #3782 ) ;
#6768=ORIENTED_EDGE ( 'NONE', *, *, #7713, .F. ) ;
#6777=DIRECTION ( 'NONE',  ( 0.000000000000000000, -0.000000000000000000, -1.000000000000000000 ) ) ;
#6797=CARTESIAN_POINT ( 'NONE',  ( -1.219727444046192735E-16, 2.000000000000000000, -5.500000000000000000 ) ) ;
#6806=DIRECTION ( 'NONE',  ( 1.000000000000000000, 0.000000000000000000, 0.000000000000000000 ) ) ;
#6827=DIRECTION ( 'NONE',  ( -0.000000000000000000, -0.000000000000000000, -1.000000000000000000 ) ) ;
#6829=AXIS2_PLACEMENT_3D ( 'NONE', #7606, #1664, #5061 ) ;
#6832=EDGE_CURVE ( 'NONE', #10839, #6057, #593, .T. ) ;
#6845=( NAMED_UNIT ( * ) PLANE_ANGLE_UNIT ( ) SI_UNIT ( $, .RADIAN. ) );
#6874=DIRECTION ( 'NONE',  ( 0.000000000000000000, 0.000000000000000000, -1.000000000000000000 ) ) ;
#6876=CIRCLE ( 'NONE', #1554, 24.99999999999999645 ) ;
#6883=ADVANCED_FACE ( 'NONE', ( #9990 ), #701, .T. ) ;
#6884=DIRECTION ( 'NONE',  ( 0.000000000000000000, 0.000000000000000000, 1.000000000000000000 ) ) ;
#6914=ORIENTED_EDGE ( 'NONE', *, *, #6607, .F. ) ;
#6917=CARTESIAN_POINT ( 'NONE',  ( -3.049318610115481714E-16, 5.000000000000000000, -2.500000000000000000 ) ) ;
#6924=LINE ( 'NONE', #5317, #8089 ) ;
#6936=DIRECTION ( 'NONE',  ( 1.000000000000000000, 6.098637220230963674E-17, 0.000000000000000000 ) ) ;
#6940=CARTESIAN_POINT ( 'NONE',  ( 29.50000000000000711, 2.000000000000001776, -12.50000000000000000 ) ) ;
#6945=DIRECTION ( 'NONE',  ( -0.000000000000000000, -0.000000000000000000, -1.000000000000000000 ) ) ;
#6948=CARTESIAN_POINT ( 'NONE',  ( 30.75045812061784289, 56.49999999999984368, 10.00000000000000178 ) ) ;
#6950=AXIS2_PLACEMENT_3D ( 'NONE', #2680, #6056, #7502 ) ;
#6951=DIRECTION ( 'NONE',  ( -1.000000000000000000, -6.098637220230963674E-17, 0.000000000000000000 ) ) ;
#6956=CARTESIAN_POINT ( 'NONE',  ( 0.000000000000000000, 0.000000000000000000, 0.000000000000000000 ) ) ;
#6957=EDGE_CURVE ( 'NONE', #874, #10104, #6277, .T. ) ;
#6961=LINE ( 'NONE', #2804, #3532 ) ;
#6962=CIRCLE ( 'NONE', #10683, 2.149999999999992362 ) ;
#6963=DIRECTION ( 'NONE',  ( 1.000000000000000000, 0.000000000000000000, 0.000000000000000000 ) ) ;
#6971=CIRCLE ( 'NONE', #2178, 4.500000000000000888 ) ;
#6979=ORIENTED_EDGE ( 'NONE', *, *, #8372, .F. ) ;
#6980=( NAMED_UNIT ( * ) PLANE_ANGLE_UNIT ( ) SI_UNIT ( $, .RADIAN. ) );
#6987=LINE ( 'NONE', #10372, #8564 ) ;
#6990=ORIENTED_EDGE ( 'NONE', *, *, #1805, .T. ) ;
#6991=CARTESIAN_POINT ( 'NONE',  ( 34.94281041931228771, 2.000000000000002220, -5.500000000000000000 ) ) ;
#6994=ORIENTED_EDGE ( 'NONE', *, *, #7524, .F. ) ;
#7016=VECTOR ( 'NONE', #8554, 1000.000000000000000 ) ;
#7018=LINE ( 'NONE', #8736, #323 ) ;
#7019=AXIS2_PLACEMENT_3D ( 'NONE', #2150, #8976, #1526 ) ;
#7032=CARTESIAN_POINT ( 'NONE',  ( 26.17691601781025312, 59.99615088301337096, 2.500000000000000000 ) ) ;
#7034=CARTESIAN_POINT ( 'NONE',  ( 21.21106610644839208, 56.49999999999984368, 10.00000000000000178 ) ) ;
#7038=EDGE_CURVE ( 'NONE', #1951, #8894, #5000, .T. ) ;
#7044=DIRECTION ( 'NONE',  ( 0.000000000000000000, 0.000000000000000000, -1.000000000000000000 ) ) ;
#7047=AXIS2_PLACEMENT_3D ( 'NONE', #8482, #8540, #1648 ) ;
#7050=EDGE_LOOP ( 'NONE', ( #5017, #8548, #5250, #8139 ) ) ;
#7054=CARTESIAN_POINT ( 'NONE',  ( 6.098637220230963427E-16, -10.00000000000000000, -10.50000000000001243 ) ) ;
#7089=CARTESIAN_POINT ( 'NONE',  ( 29.50000000000000711, 1.000000000000000888, -11.50000000000000711 ) ) ;
#7090=VERTEX_POINT ( 'NONE', #3384 ) ;
#7103=VERTEX_POINT ( 'NONE', #5329 ) ;
#7106=VERTEX_POINT ( 'NONE', #6991 ) ;
#7109=LINE ( 'NONE', #2116, #8423 ) ;
#7111=ORIENTED_EDGE ( 'NONE', *, *, #6530, .T. ) ;
#7125=LINE ( 'NONE', #1237, #6120 ) ;
#7135=DIRECTION ( 'NONE',  ( -0.000000000000000000, 1.000000000000000000, -0.000000000000000000 ) ) ;
#7145=DIRECTION ( 'NONE',  ( 6.098637220230963674E-17, -1.000000000000000000, 0.000000000000000000 ) ) ;
#7155=EDGE_LOOP ( 'NONE', ( #9714, #7327, #4427, #1816 ) ) ;
#7169=EDGE_CURVE ( 'NONE', #3195, #3312, #5440, .T. ) ;
#7170=EDGE_CURVE ( 'NONE', #1493, #7309, #9593, .T. ) ;
#7188=CARTESIAN_POINT ( 'NONE',  ( -2.649999999999885780, 30.00000000000000000, -2.500000000000000000 ) ) ;
#7189=VECTOR ( 'NONE', #2894, 1000.000000000000000 ) ;
#7190=LINE ( 'NONE', #4486, #4238 ) ;
#7219=CARTESIAN_POINT ( 'NONE',  ( -4.379688272585405606, 36.08837668307224789, 2.500000000000000000 ) ) ;
#7223=AXIS2_PLACEMENT_3D ( 'NONE', #8793, #290, #6234 ) ;
#7225=PRODUCT_DEFINITION_FORMATION_WITH_SPECIFIED_SOURCE ( 'ANY', '', #5290, .NOT_KNOWN. ) ;
#7230=VECTOR ( 'NONE', #8679, 1000.000000000000000 ) ;
#7235=ORIENTED_EDGE ( 'NONE', *, *, #5390, .T. ) ;
#7245=PLANE ( 'NONE',  #3657 ) ;
#7262=DIRECTION ( 'NONE',  ( -0.000000000000000000, 0.000000000000000000, 1.000000000000000000 ) ) ;
#7268=ORIENTED_EDGE ( 'NONE', *, *, #7170, .T. ) ;
#7278=CARTESIAN_POINT ( 'NONE',  ( 29.50000000000000711, 5.000000000000001776, 5.500000000000000000 ) ) ;
#7281=DIRECTION ( 'NONE',  ( 6.098637220230963674E-17, -1.000000000000000000, 0.000000000000000000 ) ) ;
#7285=EDGE_CURVE ( 'NONE', #8126, #3122, #6476, .T. ) ;
#7287=EDGE_CURVE ( 'NONE', #7090, #1840, #1133, .T. ) ;
#7288=AXIS2_PLACEMENT_3D ( 'NONE', #6519, #633, #8356 ) ;
#7293=DIRECTION ( 'NONE',  ( -0.000000000000000000, -0.000000000000000000, -1.000000000000000000 ) ) ;
#7309=VERTEX_POINT ( 'NONE', #6423 ) ;
#7311=VECTOR ( 'NONE', #9376, 1000.000000000000000 ) ;
#7312=CARTESIAN_POINT ( 'NONE',  ( 25.98076211353324183, 54.99999999999984368, -2.500000000000000000 ) ) ;
#7327=ORIENTED_EDGE ( 'NONE', *, *, #7170, .F. ) ;
#7339=VECTOR ( 'NONE', #5813, 1000.000000000000000 ) ;
#7348=VERTEX_POINT ( 'NONE', #3097 ) ;
#7354=DIRECTION ( 'NONE',  ( -1.000000000000000000, -6.098637220230963674E-17, 0.000000000000000000 ) ) ;
#7357=CARTESIAN_POINT ( 'NONE',  ( 30.75045812061784289, 53.49999999999983658, 14.50000000000000000 ) ) ;
#7359=CARTESIAN_POINT ( 'NONE',  ( 34.93845944406324122, 2.080102445711407011, 4.707808283735069210 ) ) ;
#7367=AXIS2_PLACEMENT_3D ( 'NONE', #5407, #7965, #9623 ) ;
#7383=CARTESIAN_POINT ( 'NONE',  ( 29.50000000000000711, -3.999999999999989786, 9.999999999999998224 ) ) ;
#7384=VECTOR ( 'NONE', #2194, 1000.000000000000000 ) ;
#7390=CARTESIAN_POINT ( 'NONE',  ( 34.94170751511534689, 2.019541143081656109, -5.105981766738329597 ) ) ;
#7395=ORIENTED_EDGE ( 'NONE', *, *, #1832, .F. ) ;
#7400=CARTESIAN_POINT ( 'NONE',  ( 34.99999999999987210, 2.000000000000002220, -12.50000000000000000 ) ) ;
#7407=CIRCLE ( 'NONE', #841, 2.649999999999991029 ) ;
#7429=EDGE_LOOP ( 'NONE', ( #6457, #1619, #6174, #7268 ) ) ;
#7438=ORIENTED_EDGE ( 'NONE', *, *, #4225, .F. ) ;
#7442=DIRECTION ( 'NONE',  ( 4.312387734422005941E-17, -0.7071067811865500152, -0.7071067811865451302 ) ) ;
#7455=LINE ( 'NONE', #8131, #1510 ) ;
#7475=EDGE_CURVE ( 'NONE', #3122, #3024, #1767, .T. ) ;
#7478=FACE_BOUND ( 'NONE', #537, .T. ) ;
#7484=VECTOR ( 'NONE', #3669, 1000.000000000000114 ) ;
#7502=DIRECTION ( 'NONE',  ( -1.000000000000000000, 0.000000000000000000, 0.000000000000000000 ) ) ;
#7515=ORIENTED_EDGE ( 'NONE', *, *, #867, .T. ) ;
#7520=CARTESIAN_POINT ( 'NONE',  ( 21.21106610644839208, 53.49999999999983658, 2.500000000000000000 ) ) ;
#7524=EDGE_CURVE ( 'NONE', #4598, #8370, #3812, .T. ) ;
#7526=CARTESIAN_POINT ( 'NONE',  ( 34.89248166448386002, 2.744837293030727210, 3.511881795860531952 ) ) ;
#7545=VERTEX_POINT ( 'NONE', #10053 ) ;
#7548=ORIENTED_EDGE ( 'NONE', *, *, #73, .F. ) ;
#7556=CARTESIAN_POINT ( 'NONE',  ( 34.99999999999987210, 1.000000000000001332, -11.50000000000000711 ) ) ;
#7559=DIRECTION ( 'NONE',  ( -0.000000000000000000, -0.000000000000000000, -1.000000000000000000 ) ) ;
#7563=ORIENTED_EDGE ( 'NONE', *, *, #3035, .T. ) ;
#7577=CYLINDRICAL_SURFACE ( 'NONE', #10251, 20.00000000000000355 ) ;
#7580=CARTESIAN_POINT ( 'NONE',  ( 21.21106610644839208, 56.49999999999984368, 2.500000000000000000 ) ) ;
#7596=PLANE ( 'NONE',  #9907 ) ;
#7605=EDGE_LOOP ( 'NONE', ( #4702, #8839, #5506, #9724, #7969, #7515 ) ) ;
#7606=CARTESIAN_POINT ( 'NONE',  ( 29.50000000000000711, -3.999999999999989786, -4.999999999999999112 ) ) ;
#7607=ORIENTED_EDGE ( 'NONE', *, *, #4082, .F. ) ;
#7609=DIRECTION ( 'NONE',  ( -0.000000000000000000, -1.000000000000000000, -0.000000000000000000 ) ) ;
#7610=VERTEX_POINT ( 'NONE', #10668 ) ;
#7650=ORIENTED_EDGE ( 'NONE', *, *, #1449, .T. ) ;
#7653=EDGE_CURVE ( 'NONE', #1662, #1634, #2283, .T. ) ;
#7658=CIRCLE ( 'NONE', #9250, 24.99999999999999645 ) ;
#7659=CARTESIAN_POINT ( 'NONE',  ( 34.99999999999987210, 16.00000000000000355, 1.499999999999902522 ) ) ;
#7670=DIRECTION ( 'NONE',  ( -1.000000000000000000, 0.000000000000000000, 0.000000000000000000 ) ) ;
#7677=CYLINDRICAL_SURFACE ( 'NONE', #6950, 30.00000000000000000 ) ;
#7679=CARTESIAN_POINT ( 'NONE',  ( 34.99999999999987210, -3.999999999999989786, -2.850000000000007194 ) ) ;
#7693=CARTESIAN_POINT ( 'NONE',  ( 25.98076211353311749, 56.49999999999984368, 10.00000000000000178 ) ) ;
#7696=B_SPLINE_CURVE_WITH_KNOTS ( 'NONE', 3,
 ( #1462, #4012, #3180, #2344, #9116, #8474, #4982, #8411, #10978, #7526, #858, #4868, #1584, #7359, #4085, #2419 ),
 .UNSPECIFIED., .F., .F.,
 ( 4, 2, 2, 2, 2, 2, 2, 4 ),
 ( 0.000000000000000000, 0.0005875779155018995932, 0.001175155831003799186, 0.001762733746505698454, 0.002350311662007598373, 0.002937889577509498074, 0.003525467493011396041, 0.004700623324015193276 ),
 .UNSPECIFIED. ) ;
#7713=EDGE_CURVE ( 'NONE', #1015, #1493, #9323, .T. ) ;
#7714=PLANE ( 'NONE',  #5548 ) ;
#7715=DIRECTION ( 'NONE',  ( -0.000000000000000000, -0.000000000000000000, -1.000000000000000000 ) ) ;
#7723=ORIENTED_EDGE ( 'NONE', *, *, #6596, .T. ) ;
#7754=CARTESIAN_POINT ( 'NONE',  ( 24.30992024302469900, 5.833333333333334814, 2.500000000000000000 ) ) ;
#7761=DIRECTION ( 'NONE',  ( 4.312387734421975126E-17, -0.7071067811865451302, -0.7071067811865500152 ) ) ;
#7789=APPLICATION_CONTEXT ( 'automotive_design' ) ;
#7793=EDGE_CURVE ( 'NONE', #1093, #2280, #5240, .T. ) ;
#7823=DIRECTION ( 'NONE',  ( 1.000000000000000000, 6.098637220230963674E-17, 0.000000000000000000 ) ) ;
#7829=ADVANCED_FACE ( 'NONE', ( #99 ), #3499, .T. ) ;
#7840=DIRECTION ( 'NONE',  ( 0.000000000000000000, 0.000000000000000000, 1.000000000000000000 ) ) ;
#7844=CARTESIAN_POINT ( 'NONE',  ( -2.649999999999887113, 30.00000000000000000, -2.500000000000000000 ) ) ;
#7862=EDGE_LOOP ( 'NONE', ( #1885, #10511 ) ) ;
#7869=CARTESIAN_POINT ( 'NONE',  ( 25.71106610644839208, 56.49999999999984368, 14.50000000000000000 ) ) ;
#7881=CARTESIAN_POINT ( 'NONE',  ( 29.17190429162964094, 2.000000000000001776, -2.500000000000000000 ) ) ;
#7883=VERTEX_POINT ( 'NONE', #1043 ) ;
#7914=FACE_OUTER_BOUND ( 'NONE', #3644, .T. ) ;
#7915=FACE_OUTER_BOUND ( 'NONE', #4612, .T. ) ;
#7936=DIRECTION ( 'NONE',  ( 0.000000000000000000, 0.000000000000000000, -1.000000000000000000 ) ) ;
#7937=CARTESIAN_POINT ( 'NONE',  ( 29.50000000000000711, 2.000000000000001776, 17.50099999999999767 ) ) ;
#7957=VERTEX_POINT ( 'NONE', #320 ) ;
#7965=DIRECTION ( 'NONE',  ( -0.000000000000000000, 1.000000000000000000, -0.000000000000000000 ) ) ;
#7969=ORIENTED_EDGE ( 'NONE', *, *, #3177, .F. ) ;
#7980=FACE_BOUND ( 'NONE', #7862, .T. ) ;
#7981=ORIENTED_EDGE ( 'NONE', *, *, #5542, .T. ) ;
#8009=ORIENTED_EDGE ( 'NONE', *, *, #6466, .F. ) ;
#8013=ADVANCED_FACE ( 'NONE', ( #263 ), #3661, .T. ) ;
#8019=CARTESIAN_POINT ( 'NONE',  ( 29.50000000000000711, 1.387778780781445676E-14, -12.50000000000000000 ) ) ;
#8023=DIRECTION ( 'NONE',  ( -1.000000000000000000, 0.000000000000000000, 0.000000000000000000 ) ) ;
#8030=FACE_BOUND ( 'NONE', #9451, .T. ) ;
#8044=CARTESIAN_POINT ( 'NONE',  ( 34.99999999999987210, -2.999999999999962252, -17.49999999999999645 ) ) ;
#8047=EDGE_CURVE ( 'NONE', #3381, #6762, #3484, .T. ) ;
#8048=DIRECTION ( 'NONE',  ( 0.000000000000000000, 0.000000000000000000, -1.000000000000000000 ) ) ;
#8067=CIRCLE ( 'NONE', #10565, 35.00000000000000000 ) ;
#8073=VECTOR ( 'NONE', #3334, 1000.000000000000114 ) ;
#8079=AXIS2_PLACEMENT_3D ( 'NONE', #5334, #1997, #8048 ) ;
#8080=CYLINDRICAL_SURFACE ( 'NONE', #4431, 5.000000000000000888 ) ;
#8089=VECTOR ( 'NONE', #1765, 1000.000000000000000 ) ;
#8090=LINE ( 'NONE', #3037, #7384 ) ;
#8098=DIRECTION ( 'NONE',  ( -0.000000000000000000, 1.000000000000000000, -0.000000000000000000 ) ) ;
#8107=EDGE_CURVE ( 'NONE', #6726, #2763, #439, .T. ) ;
#8124=CARTESIAN_POINT ( 'NONE',  ( 34.66939463810009414, 4.803388076618548830, -2.500000000000000444 ) ) ;
#8126=VERTEX_POINT ( 'NONE', #861 ) ;
#8131=CARTESIAN_POINT ( 'NONE',  ( 21.21106610644839208, 53.49999999999983658, 10.00000000000000178 ) ) ;
#8132=DIRECTION ( 'NONE',  ( 0.000000000000000000, 0.000000000000000000, 1.000000000000000000 ) ) ;
#8135=DIRECTION ( 'NONE',  ( -1.000000000000000000, 0.000000000000000000, 0.000000000000000000 ) ) ;
#8139=ORIENTED_EDGE ( 'NONE', *, *, #7038, .T. ) ;
#8151=ORIENTED_EDGE ( 'NONE', *, *, #5387, .T. ) ;
#8162=VERTEX_POINT ( 'NONE', #8536 ) ;
#8184=DIRECTION ( 'NONE',  ( 1.000000000000000000, 0.000000000000000000, 0.000000000000000000 ) ) ;
#8187=ORIENTED_EDGE ( 'NONE', *, *, #7285, .F. ) ;
#8192=DIRECTION ( 'NONE',  ( 6.098637220230963674E-17, -1.000000000000000000, 0.000000000000000000 ) ) ;
#8219=CARTESIAN_POINT ( 'NONE',  ( 34.86967549602667304, 3.020777328503462034, -3.237032597732066197 ) ) ;
#8225=AXIS2_PLACEMENT_3D ( 'NONE', #7312, #7262, #529 ) ;
#8251=ADVANCED_FACE ( 'NONE', ( #1782 ), #8553, .F. ) ;
#8256=EDGE_CURVE ( 'NONE', #10104, #1107, #209, .T. ) ;
#8258=CIRCLE ( 'NONE', #100, 4.999999999999997335 ) ;
#8275=DIRECTION ( 'NONE',  ( -1.000000000000000000, -6.098637220230963674E-17, 0.000000000000000000 ) ) ;
#8278=DIRECTION ( 'NONE',  ( -1.000000000000000000, 0.000000000000000000, -0.000000000000000000 ) ) ;
#8287=DIRECTION ( 'NONE',  ( 0.000000000000000000, 0.000000000000000000, 1.000000000000000000 ) ) ;
#8306=COLOUR_RGB ( '', 0.72549020, 0.75294118, 0.79215686) ;
#8308=EDGE_LOOP ( 'NONE', ( #3131, #10612, #1855, #9766 ) ) ;
#8312=ADVANCED_FACE ( 'NONE', ( #9491 ), #1892, .T. ) ;
#8319=EDGE_CURVE ( 'NONE', #2261, #4849, #86, .T. ) ;
#8334=FACE_OUTER_BOUND ( 'NONE', #1295, .T. ) ;
#8335=PRODUCT_DEFINITION_CONTEXT ( 'detailed design', #10047, 'design' ) ;
#8343=CYLINDRICAL_SURFACE ( 'NONE', #10096, 2.649999999999991029 ) ;
#8347=DIRECTION ( 'NONE',  ( -6.098637220230963674E-17, 1.000000000000000000, 0.000000000000000000 ) ) ;
#8356=DIRECTION ( 'NONE',  ( 0.000000000000000000, 0.000000000000000000, -1.000000000000000000 ) ) ;
#8359=LINE ( 'NONE', #5039, #6309 ) ;
#8363=FACE_OUTER_BOUND ( 'NONE', #2916, .T. ) ;
#8369=CIRCLE ( 'NONE', #2714, 2.149999999999992362 ) ;
#8370=VERTEX_POINT ( 'NONE', #6263 ) ;
#8372=EDGE_CURVE ( 'NONE', #10564, #7610, #1149, .T. ) ;
#8375=CARTESIAN_POINT ( 'NONE',  ( 21.21106610644839208, 53.49999999999983658, 2.500000000000000000 ) ) ;
#8377=ORIENTED_EDGE ( 'NONE', *, *, #10764, .F. ) ;
#8378=DIRECTION ( 'NONE',  ( 1.000000000000000000, 0.000000000000000000, 0.000000000000000000 ) ) ;
#8382=DIRECTION ( 'NONE',  ( -0.000000000000000000, -0.000000000000000000, -1.000000000000000000 ) ) ;
#8391=CARTESIAN_POINT ( 'NONE',  ( 29.50000000000000711, 2.000000000000001776, -12.50000000000000000 ) ) ;
#8401=LINE ( 'NONE', #3356, #1682 ) ;
#8411=CARTESIAN_POINT ( 'NONE',  ( 34.85586774767502760, 3.177316488306996423, 3.109148447068123655 ) ) ;
#8413=AXIS2_PLACEMENT_3D ( 'NONE', #5935, #6884, #2670 ) ;
#8423=VECTOR ( 'NONE', #1156, 1000.000000000000000 ) ;
#8424=CIRCLE ( 'NONE', #10025, 30.00000000000000000 ) ;
#8447=EDGE_CURVE ( 'NONE', #9319, #6022, #9552, .T. ) ;
#8471=CIRCLE ( 'NONE', #2445, 2.649999999999991029 ) ;
#8474=CARTESIAN_POINT ( 'NONE',  ( 34.80692069235085029, 3.675807134350210337, 2.800930295893637734 ) ) ;
#8476=EDGE_CURVE ( 'NONE', #3879, #7957, #3822, .T. ) ;
#8482=CARTESIAN_POINT ( 'NONE',  ( 24.99999259214812142, 30.01924558493218598, 2.500000000000000000 ) ) ;
#8487=DIRECTION ( 'NONE',  ( -1.000000000000000000, 2.212882687011047826E-16, 0.000000000000000000 ) ) ;
#8498=CARTESIAN_POINT ( 'NONE',  ( 0.000000000000000000, 0.000000000000000000, 2.500000000000000000 ) ) ;
#8506=DIRECTION ( 'NONE',  ( 1.000000000000000000, -9.251858538542971828E-16, 0.000000000000000000 ) ) ;
#8516=( NAMED_UNIT ( * ) SI_UNIT ( $, .STERADIAN. ) SOLID_ANGLE_UNIT ( ) );
#8518=DIRECTION ( 'NONE',  ( -0.000000000000000000, 0.000000000000000000, 1.000000000000000000 ) ) ;
#8525=VERTEX_POINT ( 'NONE', #1154 ) ;
#8529=LINE ( 'NONE', #7580, #1167 ) ;
#8536=CARTESIAN_POINT ( 'NONE',  ( 26.25045812061784289, 56.49999999999984368, 14.50000000000000000 ) ) ;
#8538=ORIENTED_EDGE ( 'NONE', *, *, #5387, .F. ) ;
#8540=DIRECTION ( 'NONE',  ( 0.000000000000000000, -0.000000000000000000, -1.000000000000000000 ) ) ;
#8547=ORIENTED_EDGE ( 'NONE', *, *, #460, .F. ) ;
#8548=ORIENTED_EDGE ( 'NONE', *, *, #10280, .T. ) ;
#8553=CYLINDRICAL_SURFACE ( 'NONE', #6297, 24.99999999999999645 ) ;
#8554=DIRECTION ( 'NONE',  ( -0.000000000000000000, 1.000000000000000000, -0.000000000000000000 ) ) ;
#8555=CARTESIAN_POINT ( 'NONE',  ( 1.047444401652940007E-13, 30.00000000000000000, 2.500000000000000000 ) ) ;
#8564=VECTOR ( 'NONE', #5496, 1000.000000000000000 ) ;
#8567=SURFACE_STYLE_USAGE ( .BOTH. , #5297 ) ;
#8587=LINE ( 'NONE', #8702, #9681 ) ;
#8596=LINE ( 'NONE', #1823, #7311 ) ;
#8627=DIRECTION ( 'NONE',  ( 1.000000000000000000, 0.000000000000000000, 0.000000000000000000 ) ) ;
#8629=VECTOR ( 'NONE', #3303, 1000.000000000000000 ) ;
#8635=ORIENTED_EDGE ( 'NONE', *, *, #632, .F. ) ;
#8643=CARTESIAN_POINT ( 'NONE',  ( 26.17691601781025312, 59.99615088301337096, -2.500000000000000000 ) ) ;
#8647=SURFACE_SIDE_STYLE ('',( #5319 ) ) ;
#8658=VECTOR ( 'NONE', #4567, 1000.000000000000000 ) ;
#8659=AXIS2_PLACEMENT_3D ( 'NONE', #2857, #6227, #4630 ) ;
#8674=CARTESIAN_POINT ( 'NONE',  ( 29.50000000000000711, 5.000000000000001776, -2.500000000000000000 ) ) ;
#8679=DIRECTION ( 'NONE',  ( 1.000000000000000000, -0.000000000000000000, -0.000000000000000000 ) ) ;
#8681=AXIS2_PLACEMENT_3D ( 'NONE', #8910, #10682, #8132 ) ;
#8690=FACE_OUTER_BOUND ( 'NONE', #7605, .T. ) ;
#8692=ADVANCED_FACE ( 'NONE', ( #9644 ), #6251, .F. ) ;
#8694=DIRECTION ( 'NONE',  ( -1.000000000000000000, 0.000000000000000000, -0.000000000000000000 ) ) ;
#8695=CARTESIAN_POINT ( 'NONE',  ( 29.50000000000000711, -3.999999999999989786, -7.149999999999991473 ) ) ;
#8701=DIRECTION ( 'NONE',  ( 1.000000000000000000, 0.000000000000000000, 0.000000000000000000 ) ) ;
#8702=CARTESIAN_POINT ( 'NONE',  ( 34.99999999999987210, -3.999999999999989786, 12.14999999999999147 ) ) ;
#8708=CARTESIAN_POINT ( 'NONE',  ( 29.50000000000000711, -3.999999999999989786, -4.999999999999999112 ) ) ;
#8719=CARTESIAN_POINT ( 'NONE',  ( 24.30992024302470256, 5.833333333333335702, 2.500000000000000000 ) ) ;
#8721=EDGE_CURVE ( 'NONE', #874, #40, #3760, .T. ) ;
#8722=DIRECTION ( 'NONE',  ( -0.000000000000000000, -1.000000000000000000, -0.000000000000000000 ) ) ;
#8736=CARTESIAN_POINT ( 'NONE',  ( 29.50000000000000711, -2.999999999999962697, -17.49999999999999645 ) ) ;
#8751=ADVANCED_FACE ( 'NONE', ( #1085 ), #8876, .T. ) ;
#8757=CARTESIAN_POINT ( 'NONE',  ( 34.99999999999987210, -3.999999999999989786, 9.999999999999998224 ) ) ;
#8768=ORIENTED_EDGE ( 'NONE', *, *, #10486, .F. ) ;
#8772=EDGE_CURVE ( 'NONE', #6022, #10302, #2755, .T. ) ;
#8793=CARTESIAN_POINT ( 'NONE',  ( 26.25045812061784289, 0.000000000000000000, 10.00000000000000178 ) ) ;
#8797=EDGE_CURVE ( 'NONE', #2763, #1093, #683, .T. ) ;
#8823=DIRECTION ( 'NONE',  ( 1.000000000000000000, -0.000000000000000000, -0.000000000000000000 ) ) ;
#8835=CIRCLE ( 'NONE', #4579, 7.500000000000000000 ) ;
#8839=ORIENTED_EDGE ( 'NONE', *, *, #2088, .T. ) ;
#8852=AXIS2_PLACEMENT_3D ( 'NONE', #454, #4804, #2139 ) ;
#8876=PLANE ( 'NONE',  #6631 ) ;
#8882=EDGE_LOOP ( 'NONE', ( #4467, #6682, #6151, #7723 ) ) ;
#8891=ADVANCED_FACE ( 'NONE', ( #2356 ), #5746, .T. ) ;
#8893=DIRECTION ( 'NONE',  ( 0.000000000000000000, 1.000000000000000000, 0.000000000000000000 ) ) ;
#8894=VERTEX_POINT ( 'NONE', #9076 ) ;
#8901=LINE ( 'NONE', #230, #2114 ) ;
#8907=DIRECTION ( 'NONE',  ( -0.000000000000000000, -0.000000000000000000, -1.000000000000000000 ) ) ;
#8910=CARTESIAN_POINT ( 'NONE',  ( 25.71106610644839208, 53.49999999999983658, 10.00000000000000178 ) ) ;
#8913=DIRECTION ( 'NONE',  ( -0.000000000000000000, -0.000000000000000000, -1.000000000000000000 ) ) ;
#8928=EDGE_LOOP ( 'NONE', ( #7438, #9769 ) ) ;
#8940=AXIS2_PLACEMENT_3D ( 'NONE', #10934, #5222, #1657 ) ;
#8950=PLANE ( 'NONE',  #5636 ) ;
#8954=CARTESIAN_POINT ( 'NONE',  ( 34.89259351528887976, 2.743407123163641437, -3.513512538347001612 ) ) ;
#8976=DIRECTION ( 'NONE',  ( -0.000000000000000000, 0.000000000000000000, 1.000000000000000000 ) ) ;
#8984=ORIENTED_EDGE ( 'NONE', *, *, #6832, .F. ) ;
#8989=VERTEX_POINT ( 'NONE', #4432 ) ;
#8999=ORIENTED_EDGE ( 'NONE', *, *, #4342, .T. ) ;
#9007=VECTOR ( 'NONE', #9733, 1000.000000000000000 ) ;
#9025=CARTESIAN_POINT ( 'NONE',  ( 0.000000000000000000, 0.000000000000000000, -2.500000000000000000 ) ) ;
#9046=ORIENTED_EDGE ( 'NONE', *, *, #9598, .T. ) ;
#9057=CARTESIAN_POINT ( 'NONE',  ( 34.93719828579780540, 2.096102678619137905, -4.721690477507365813 ) ) ;
#9070=CARTESIAN_POINT ( 'NONE',  ( 34.99999999999987210, 2.000000000000002220, -12.50000000000000000 ) ) ;
#9076=CARTESIAN_POINT ( 'NONE',  ( 21.21106610644839208, 53.49999999999983658, 2.500000000000000000 ) ) ;
#9082=DIRECTION ( 'NONE',  ( -0.000000000000000000, -0.000000000000000000, -1.000000000000000000 ) ) ;
#9108=VERTEX_POINT ( 'NONE', #9996 ) ;
#9110=VERTEX_POINT ( 'NONE', #6595 ) ;
#9116=CARTESIAN_POINT ( 'NONE',  ( 34.76670834929980458, 4.038474554490624868, 2.651503408690715435 ) ) ;
#9118=AXIS2_PLACEMENT_3D ( 'NONE', #8757, #5323, #7044 ) ;
#9129=AXIS2_PLACEMENT_3D ( 'NONE', #5155, #5316, #8701 ) ;
#9132=ADVANCED_FACE ( 'NONE', ( #9217 ), #1610, .T. ) ;
#9149=EDGE_CURVE ( 'NONE', #7883, #5054, #4160, .T. ) ;
#9158=VECTOR ( 'NONE', #4586, 1000.000000000000000 ) ;
#9166=ORIENTED_EDGE ( 'NONE', *, *, #1354, .T. ) ;
#9179=FACE_BOUND ( 'NONE', #5146, .T. ) ;
#9188=DIRECTION ( 'NONE',  ( -0.000000000000000000, -0.000000000000000000, -1.000000000000000000 ) ) ;
#9194=VECTOR ( 'NONE', #4321, 1000.000000000000000 ) ;
#9208=VERTEX_POINT ( 'NONE', #1835 ) ;
#9214=ORIENTED_EDGE ( 'NONE', *, *, #3560, .F. ) ;
#9217=FACE_OUTER_BOUND ( 'NONE', #3000, .T. ) ;
#9220=EDGE_CURVE ( 'NONE', #7610, #9110, #3504, .T. ) ;
#9238=CARTESIAN_POINT ( 'NONE',  ( 34.99999999999987210, -3.999999999999989786, -4.999999999999999112 ) ) ;
#9244=CARTESIAN_POINT ( 'NONE',  ( 25.98076211353324183, 54.99999999999984368, 2.500000000000000000 ) ) ;
#9250=AXIS2_PLACEMENT_3D ( 'NONE', #9277, #6777, #53 ) ;
#9273=EDGE_CURVE ( 'NONE', #750, #7348, #786, .T. ) ;
#9277=CARTESIAN_POINT ( 'NONE',  ( 0.000000000000000000, 0.000000000000000000, 2.500000000000000000 ) ) ;
#9284=EDGE_CURVE ( 'NONE', #6429, #4729, #5282, .T. ) ;
#9286=DIRECTION ( 'NONE',  ( 1.000000000000000000, -5.319818659662208633E-14, 0.000000000000000000 ) ) ;
#9293=EDGE_LOOP ( 'NONE', ( #6717, #5704, #1563, #7650 ) ) ;
#9294=FACE_OUTER_BOUND ( 'NONE', #6327, .T. ) ;
#9301=CARTESIAN_POINT ( 'NONE',  ( 25.71106610644839208, 0.000000000000000000, 10.00000000000000178 ) ) ;
#9319=VERTEX_POINT ( 'NONE', #9386 ) ;
#9323=LINE ( 'NONE', #9381, #5930 ) ;
#9339=ORIENTED_EDGE ( 'NONE', *, *, #3701, .F. ) ;
#9340=PLANE ( 'NONE',  #1018 ) ;
#9341=ORIENTED_EDGE ( 'NONE', *, *, #920, .F. ) ;
#9352=LINE ( 'NONE', #4249, #2392 ) ;
#9357=LINE ( 'NONE', #7520, #8629 ) ;
#9371=CARTESIAN_POINT ( 'NONE',  ( 25.98076211353324183, 54.99999999999984368, 2.500000000000000000 ) ) ;
#9376=DIRECTION ( 'NONE',  ( -0.000000000000000000, -0.000000000000000000, -1.000000000000000000 ) ) ;
#9381=CARTESIAN_POINT ( 'NONE',  ( 29.50000000000000711, 2.000000000000001776, 17.49999999999999645 ) ) ;
#9386=CARTESIAN_POINT ( 'NONE',  ( 29.50000000000000711, 5.000000000000001776, 2.500000000000000000 ) ) ;
#9405=CARTESIAN_POINT ( 'NONE',  ( 34.64101615137754919, 5.000000000000002665, 2.500000000000000000 ) ) ;
#9406=ORIENTED_EDGE ( 'NONE', *, *, #4225, .T. ) ;
#9409=EDGE_CURVE ( 'NONE', #10935, #1662, #7109, .T. ) ;
#9413=DIRECTION ( 'NONE',  ( -0.000000000000000000, 0.000000000000000000, 1.000000000000000000 ) ) ;
#9417=DIRECTION ( 'NONE',  ( -0.000000000000000000, -0.000000000000000000, -1.000000000000000000 ) ) ;
#9441=CARTESIAN_POINT ( 'NONE',  ( 29.50000000000000711, 16.00000000000000000, 1.499999999999902522 ) ) ;
#9451=EDGE_LOOP ( 'NONE', ( #3836, #9341 ) ) ;
#9461=ORIENTED_EDGE ( 'NONE', *, *, #98, .T. ) ;
#9462=ORIENTED_EDGE ( 'NONE', *, *, #10489, .F. ) ;
#9473=DIRECTION ( 'NONE',  ( -0.000000000000000000, -0.000000000000000000, -1.000000000000000000 ) ) ;
#9488=DIRECTION ( 'NONE',  ( 0.000000000000000000, -0.000000000000000000, -1.000000000000000000 ) ) ;
#9491=FACE_OUTER_BOUND ( 'NONE', #7155, .T. ) ;
#9528=DIRECTION ( 'NONE',  ( -0.000000000000000000, -0.000000000000000000, -1.000000000000000000 ) ) ;
#9550=ORIENTED_EDGE ( 'NONE', *, *, #3563, .T. ) ;
#9552=LINE ( 'NONE', #1325, #7189 ) ;
#9556=CARTESIAN_POINT ( 'NONE',  ( 26.25045812061784289, 53.49999999999983658, 10.00000000000000178 ) ) ;
#9563=ORIENTED_EDGE ( 'NONE', *, *, #8447, .T. ) ;
#9565=DIRECTION ( 'NONE',  ( 1.000000000000000000, 0.000000000000000000, 0.000000000000000000 ) ) ;
#9587=DIRECTION ( 'NONE',  ( -0.000000000000000000, 0.000000000000000000, 1.000000000000000000 ) ) ;
#9593=LINE ( 'NONE', #6095, #2200 ) ;
#9598=EDGE_CURVE ( 'NONE', #3312, #10201, #5947, .T. ) ;
#9618=CARTESIAN_POINT ( 'NONE',  ( 29.50000000000000711, -17.99999999999996803, 7.500000000000038192 ) ) ;
#9623=DIRECTION ( 'NONE',  ( 0.000000000000000000, 0.000000000000000000, -1.000000000000000000 ) ) ;
#9627=DIRECTION ( 'NONE',  ( 1.000000000000000000, -2.212882687011047826E-16, 0.000000000000000000 ) ) ;
#9634=DIRECTION ( 'NONE',  ( 1.000000000000000000, 8.881784197001252323E-16, 0.000000000000000000 ) ) ;
#9638=CARTESIAN_POINT ( 'NONE',  ( -4.379688272585402942, 36.08837668307224789, 0.000000000000000000 ) ) ;
#9644=FACE_OUTER_BOUND ( 'NONE', #1575, .T. ) ;
#9651=ADVANCED_FACE ( 'NONE', ( #4710 ), #1141, .F. ) ;
#9652=ORIENTED_EDGE ( 'NONE', *, *, #2056, .T. ) ;
#9659=AXIS2_PLACEMENT_3D ( 'NONE', #9866, #6621, #5697 ) ;
#9681=VECTOR ( 'NONE', #3698, 1000.000000000000000 ) ;
#9714=ORIENTED_EDGE ( 'NONE', *, *, #98, .F. ) ;
#9718=AXIS2_PLACEMENT_3D ( 'NONE', #7278, #5623, #10718 ) ;
#9722=ORIENTED_EDGE ( 'NONE', *, *, #524, .T. ) ;
#9723=DIRECTION ( 'NONE',  ( 1.000000000000000000, -0.000000000000000000, -0.000000000000000000 ) ) ;
#9724=ORIENTED_EDGE ( 'NONE', *, *, #4241, .T. ) ;
#9733=DIRECTION ( 'NONE',  ( -4.312387734421997929E-17, 0.7071067811865487940, 0.7071067811865463515 ) ) ;
#9741=ORIENTED_EDGE ( 'NONE', *, *, #6832, .T. ) ;
#9744=FACE_OUTER_BOUND ( 'NONE', #3784, .T. ) ;
#9746=CARTESIAN_POINT ( 'NONE',  ( 29.50000000000000711, -9.999999999999998224, 15.49999999999998934 ) ) ;
#9766=ORIENTED_EDGE ( 'NONE', *, *, #8797, .F. ) ;
#9769=ORIENTED_EDGE ( 'NONE', *, *, #1202, .F. ) ;
#9777=DIRECTION ( 'NONE',  ( -0.000000000000000000, 0.000000000000000000, 1.000000000000000000 ) ) ;
#9800=ADVANCED_FACE ( 'NONE', ( #3967 ), #684, .F. ) ;
#9803=DIRECTION ( 'NONE',  ( -1.000000000000000000, -6.098637220230963674E-17, 0.000000000000000000 ) ) ;
#9804=VERTEX_POINT ( 'NONE', #2196 ) ;
#9840=CYLINDRICAL_SURFACE ( 'NONE', #5463, 2.149999999999992362 ) ;
#9847=ORIENTED_EDGE ( 'NONE', *, *, #4082, .T. ) ;
#9853=AXIS2_PLACEMENT_3D ( 'NONE', #10471, #4638, #2918 ) ;
#9856=FACE_OUTER_BOUND ( 'NONE', #10006, .T. ) ;
#9860=EDGE_LOOP ( 'NONE', ( #1635, #506 ) ) ;
#9866=CARTESIAN_POINT ( 'NONE',  ( 3.469446951953614189E-15, -1.040834085586084257E-14, 2.500000000000000000 ) ) ;
#9907=AXIS2_PLACEMENT_3D ( 'NONE', #10867, #4207, #5921 ) ;
#9911=CARTESIAN_POINT ( 'NONE',  ( 0.000000000000000000, 30.00000000000000000, -2.499999999999998668 ) ) ;
#9952=CARTESIAN_POINT ( 'NONE',  ( 34.80704760714191082, 3.674543421742910709, -2.801642449272108593 ) ) ;
#9977=ORIENTED_EDGE ( 'NONE', *, *, #7287, .T. ) ;
#9990=FACE_OUTER_BOUND ( 'NONE', #7429, .T. ) ;
#9996=CARTESIAN_POINT ( 'NONE',  ( 30.75045812061784289, 53.49999999999983658, 10.00000000000000178 ) ) ;
#10001=CARTESIAN_POINT ( 'NONE',  ( 29.50000000000000711, 1.799097979968134709E-15, 2.500000000000000000 ) ) ;
#10006=EDGE_LOOP ( 'NONE', ( #8768, #1134, #10534, #247 ) ) ;
#10018=PLANE ( 'NONE',  #3639 ) ;
#10020=ORIENTED_EDGE ( 'NONE', *, *, #4597, .F. ) ;
#10023=AXIS2_PLACEMENT_3D ( 'NONE', #5227, #6827, #10170 ) ;
#10025=AXIS2_PLACEMENT_3D ( 'NONE', #10888, #3280, #8506 ) ;
#10047=APPLICATION_CONTEXT ( 'automotive_design' ) ;
#10053=CARTESIAN_POINT ( 'NONE',  ( 2.650000000000095834, 30.00000000000000000, 2.500000000000000000 ) ) ;
#10066=AXIS2_PLACEMENT_3D ( 'NONE', #8019, #391, #2914 ) ;
#10083=( GEOMETRIC_REPRESENTATION_CONTEXT ( 3 ) GLOBAL_UNCERTAINTY_ASSIGNED_CONTEXT ( ( #1436 ) ) GLOBAL_UNIT_ASSIGNED_CONTEXT ( ( #6013, #6845, #8516 ) ) REPRESENTATION_CONTEXT ( 'NONE', 'WORKASPACE' ) );
#10093=CARTESIAN_POINT ( 'NONE',  ( 30.75045812061784289, 56.49999999999984368, 2.500000000000000000 ) ) ;
#10096=AXIS2_PLACEMENT_3D ( 'NONE', #6561, #4183, #3352 ) ;
#10104=VERTEX_POINT ( 'NONE', #6293 ) ;
#10132=DIRECTION ( 'NONE',  ( -0.000000000000000000, 1.000000000000000000, -0.000000000000000000 ) ) ;
#10135=EDGE_LOOP ( 'NONE', ( #1993, #2204, #5929, #2710 ) ) ;
#10143=FACE_OUTER_BOUND ( 'NONE', #9293, .T. ) ;
#10151=FACE_BOUND ( 'NONE', #4784, .T. ) ;
#10153=EDGE_CURVE ( 'NONE', #1456, #10839, #2023, .T. ) ;
#10160=ORIENTED_EDGE ( 'NONE', *, *, #2542, .T. ) ;
#10163=ORIENTED_EDGE ( 'NONE', *, *, #10486, .T. ) ;
#10170=DIRECTION ( 'NONE',  ( -1.000000000000000000, 0.000000000000000000, 0.000000000000000000 ) ) ;
#10186=CARTESIAN_POINT ( 'NONE',  ( 3.469446951953614189E-15, -1.040834085586084257E-14, -2.500000000000000000 ) ) ;
#10201=VERTEX_POINT ( 'NONE', #7032 ) ;
#10204=VECTOR ( 'NONE', #9417, 1000.000000000000000 ) ;
#10231=FACE_OUTER_BOUND ( 'NONE', #916, .T. ) ;
#10234=ORIENTED_EDGE ( 'NONE', *, *, #9409, .F. ) ;
#10249=CARTESIAN_POINT ( 'NONE',  ( 25.98076211353311749, 56.49999999999984368, 10.00000000000000178 ) ) ;
#10251=AXIS2_PLACEMENT_3D ( 'NONE', #4018, #5793, #4077 ) ;
#10280=EDGE_CURVE ( 'NONE', #10997, #10983, #7455, .T. ) ;
#10291=ORIENTED_EDGE ( 'NONE', *, *, #1402, .F. ) ;
#10293=FILL_AREA_STYLE_COLOUR ( '', #842 ) ;
#10300=CARTESIAN_POINT ( 'NONE',  ( 21.21106610644839208, 53.49999999999983658, 14.50000000000000000 ) ) ;
#10302=VERTEX_POINT ( 'NONE', #4913 ) ;
#10338=ORIENTED_EDGE ( 'NONE', *, *, #3531, .T. ) ;
#10341=ORIENTED_EDGE ( 'NONE', *, *, #500, .T. ) ;
#10354=ORIENTED_EDGE ( 'NONE', *, *, #10658, .T. ) ;
#10367=SURFACE_STYLE_USAGE ( .BOTH. , #8647 ) ;
#10372=CARTESIAN_POINT ( 'NONE',  ( -1.219727444046192735E-16, 2.000000000000000000, 15.49999999999999645 ) ) ;
#10396=EDGE_LOOP ( 'NONE', ( #2584, #10291, #5030, #10830 ) ) ;
#10401=DIRECTION ( 'NONE',  ( 0.000000000000000000, 0.000000000000000000, 1.000000000000000000 ) ) ;
#10435=EDGE_CURVE ( 'NONE', #4729, #2494, #8258, .T. ) ;
#10450=VECTOR ( 'NONE', #9528, 1000.000000000000000 ) ;
#10457=CARTESIAN_POINT ( 'NONE',  ( 34.99999999999987210, -3.999999999999989786, -7.149999999999991473 ) ) ;
#10471=CARTESIAN_POINT ( 'NONE',  ( 0.000000000000000000, 0.000000000000000000, 2.500000000000000000 ) ) ;
#10476=LINE ( 'NONE', #7188, #2806 ) ;
#10486=EDGE_CURVE ( 'NONE', #1437, #6429, #6699, .T. ) ;
#10487=CARTESIAN_POINT ( 'NONE',  ( 29.50000000000000711, 1.799097979968134709E-15, -2.500000000000000000 ) ) ;
#10489=EDGE_CURVE ( 'NONE', #10302, #3381, #8835, .T. ) ;
#10502=EDGE_CURVE ( 'NONE', #10839, #1493, #2800, .T. ) ;
#10511=ORIENTED_EDGE ( 'NONE', *, *, #1354, .F. ) ;
#10523=EDGE_LOOP ( 'NONE', ( #9741, #1057, #3794, #3963 ) ) ;
#10524=CARTESIAN_POINT ( 'NONE',  ( 25.58039891549807976, 2.000000000000002665, -2.500000000000000000 ) ) ;
#10534=ORIENTED_EDGE ( 'NONE', *, *, #10435, .F. ) ;
#10535=DIRECTION ( 'NONE',  ( 6.098637220230963674E-17, -1.000000000000000000, 0.000000000000000000 ) ) ;
#10564=VERTEX_POINT ( 'NONE', #4417 ) ;
#10565=AXIS2_PLACEMENT_3D ( 'NONE', #10186, #2644, #6963 ) ;
#10575=FACE_OUTER_BOUND ( 'NONE', #10632, .T. ) ;
#10576=ORIENTED_EDGE ( 'NONE', *, *, #3580, .F. ) ;
#10577=ORIENTED_EDGE ( 'NONE', *, *, #498, .F. ) ;
#10587=CARTESIAN_POINT ( 'NONE',  ( 25.78460820925620922, 50.00384911698630930, 2.500000000000000000 ) ) ;
#10589=PLANE ( 'NONE',  #2412 ) ;
#10612=ORIENTED_EDGE ( 'NONE', *, *, #3701, .T. ) ;
#10614=EDGE_LOOP ( 'NONE', ( #6208, #5681 ) ) ;
#10615=DIRECTION ( 'NONE',  ( -0.000000000000000000, 0.000000000000000000, 1.000000000000000000 ) ) ;
#10623=ADVANCED_FACE ( 'NONE', ( #4518 ), #9840, .F. ) ;
#10632=EDGE_LOOP ( 'NONE', ( #10576, #6329, #679, #10020 ) ) ;
#10644=DIRECTION ( 'NONE',  ( 0.000000000000000000, -0.000000000000000000, -1.000000000000000000 ) ) ;
#10655=ORIENTED_EDGE ( 'NONE', *, *, #6338, .F. ) ;
#10658=EDGE_CURVE ( 'NONE', #9804, #9319, #658, .T. ) ;
#10668=CARTESIAN_POINT ( 'NONE',  ( 25.98076211353311749, 53.49999999999983658, 12.14999999999999147 ) ) ;
#10682=DIRECTION ( 'NONE',  ( -0.000000000000000000, -1.000000000000000000, -0.000000000000000000 ) ) ;
#10683=AXIS2_PLACEMENT_3D ( 'NONE', #8708, #6149, #1315 ) ;
#10689=ORIENTED_EDGE ( 'NONE', *, *, #4597, .T. ) ;
#10690=ADVANCED_FACE ( 'NONE', ( #6551 ), #8950, .F. ) ;
#10694=CARTESIAN_POINT ( 'NONE',  ( 29.50000000000000711, -3.999999999999989786, 7.850000000000005862 ) ) ;
#10701=ORIENTED_EDGE ( 'NONE', *, *, #4819, .T. ) ;
#10703=DIRECTION ( 'NONE',  ( -4.312387734422005941E-17, 0.7071067811865500152, -0.7071067811865451302 ) ) ;
#10708=EDGE_LOOP ( 'NONE', ( #6914, #8377 ) ) ;
#10710=AXIS2_PLACEMENT_3D ( 'NONE', #4102, #9777, #2169 ) ;
#10718=DIRECTION ( 'NONE',  ( 0.000000000000000000, -1.000000000000000000, 0.000000000000000000 ) ) ;
#10723=DIRECTION ( 'NONE',  ( -0.000000000000000000, -0.000000000000000000, -1.000000000000000000 ) ) ;
#10725=CLOSED_SHELL ( 'NONE', ( #9651, #4932, #8692, #10623, #4866, #3759, #8891, #5826, #9132, #565, #8251, #4654, #23, #377, #5022, #6883, #8751, #6450, #8013, #6141, #10690, #8312, #4519, #5193, #7829, #1954, #9800, #3696, #4489, #6014, #4386, #1753, #6074, #6350, #2435, #2211, #4166, #1104, #1937 ) ) ;
#10732=CIRCLE ( 'NONE', #4184, 2.149999999999992362 ) ;
#10738=FACE_OUTER_BOUND ( 'NONE', #3994, .T. ) ;
#10764=EDGE_CURVE ( 'NONE', #7545, #8989, #8471, .T. ) ;
#10769=ORIENTED_EDGE ( 'NONE', *, *, #2542, .F. ) ;
#10783=CARTESIAN_POINT ( 'NONE',  ( 34.90224802882305255, 2.616310811731261676, -3.667896704194531843 ) ) ;
#10784=CARTESIAN_POINT ( 'NONE',  ( 34.99999999999987210, -3.999999999999989786, -4.999999999999999112 ) ) ;
#10799=B_SPLINE_CURVE_WITH_KNOTS ( 'NONE', 3,
 ( #3068, #1404, #7390, #9057, #4845, #5573, #2179, #10783, #8954, #8219, #6554, #606, #9952, #2336, #5780, #1503, #8124, #4905 ),
 .UNSPECIFIED., .F., .F.,
 ( 4, 2, 2, 2, 2, 2, 2, 2, 4 ),
 ( 0.000000000000000000, 0.0005875687307069781158, 0.001175137461413956232, 0.001762706192120934131, 0.002350274922827913331, 0.002937843653534892747, 0.003525412384241871731, 0.004112981114948850714, 0.004700549845655830131 ),
 .UNSPECIFIED. ) ;
#10802=CARTESIAN_POINT ( 'NONE',  ( 29.50000000000000711, 1.387778780781445676E-14, -12.50000000000000000 ) ) ;
#10828=DIRECTION ( 'NONE',  ( -1.000000000000000000, -6.098637220230963674E-17, 0.000000000000000000 ) ) ;
#10830=ORIENTED_EDGE ( 'NONE', *, *, #823, .F. ) ;
#10839=VERTEX_POINT ( 'NONE', #6721 ) ;
#10845=FACE_OUTER_BOUND ( 'NONE', #5134, .T. ) ;
#10851=ORIENTED_EDGE ( 'NONE', *, *, #3177, .T. ) ;
#10867=CARTESIAN_POINT ( 'NONE',  ( 29.50000000000000711, 2.000000000000001776, -12.50000000000000000 ) ) ;
#10872=EDGE_LOOP ( 'NONE', ( #8635, #66, #156, #10234 ) ) ;
#10874=ORIENTED_EDGE ( 'NONE', *, *, #632, .T. ) ;
#10876=DIRECTION ( 'NONE',  ( -0.000000000000000000, -0.000000000000000000, -1.000000000000000000 ) ) ;
#10888=CARTESIAN_POINT ( 'NONE',  ( 24.99999259214812142, 30.01924558493218598, -2.500000000000000000 ) ) ;
#10892=ORIENTED_EDGE ( 'NONE', *, *, #1324, .F. ) ;
#10896=AXIS2_PLACEMENT_3D ( 'NONE', #7383, #10828, #3940 ) ;
#10897=EDGE_CURVE ( 'NONE', #1093, #6429, #6876, .T. ) ;
#10916=CYLINDRICAL_SURFACE ( 'NONE', #7288, 2.149999999999992362 ) ;
#10927=CIRCLE ( 'NONE', #992, 2.149999999999994582 ) ;
#10933=EDGE_LOOP ( 'NONE', ( #6979, #6990, #9166, #4319 ) ) ;
#10934=CARTESIAN_POINT ( 'NONE',  ( 29.50000000000000711, 5.000000000000001776, -5.500000000000000000 ) ) ;
#10935=VERTEX_POINT ( 'NONE', #7869 ) ;
#10941=EDGE_CURVE ( 'NONE', #8989, #750, #10476, .T. ) ;
#10965=CARTESIAN_POINT ( 'NONE',  ( 29.50000000000000711, 2.000000000000001776, -2.500000000000000000 ) ) ;
#10978=CARTESIAN_POINT ( 'NONE',  ( 34.86952523334976917, 3.022518564432433941, 3.235504471074991617 ) ) ;
#10983=VERTEX_POINT ( 'NONE', #7034 ) ;
#10985=CARTESIAN_POINT ( 'NONE',  ( 34.99999999999987210, -9.999999999999998224, -12.50000000000000000 ) ) ;
#10997=VERTEX_POINT ( 'NONE', #4592 ) ;
ENDSEC;
END-ISO-10303-21;
